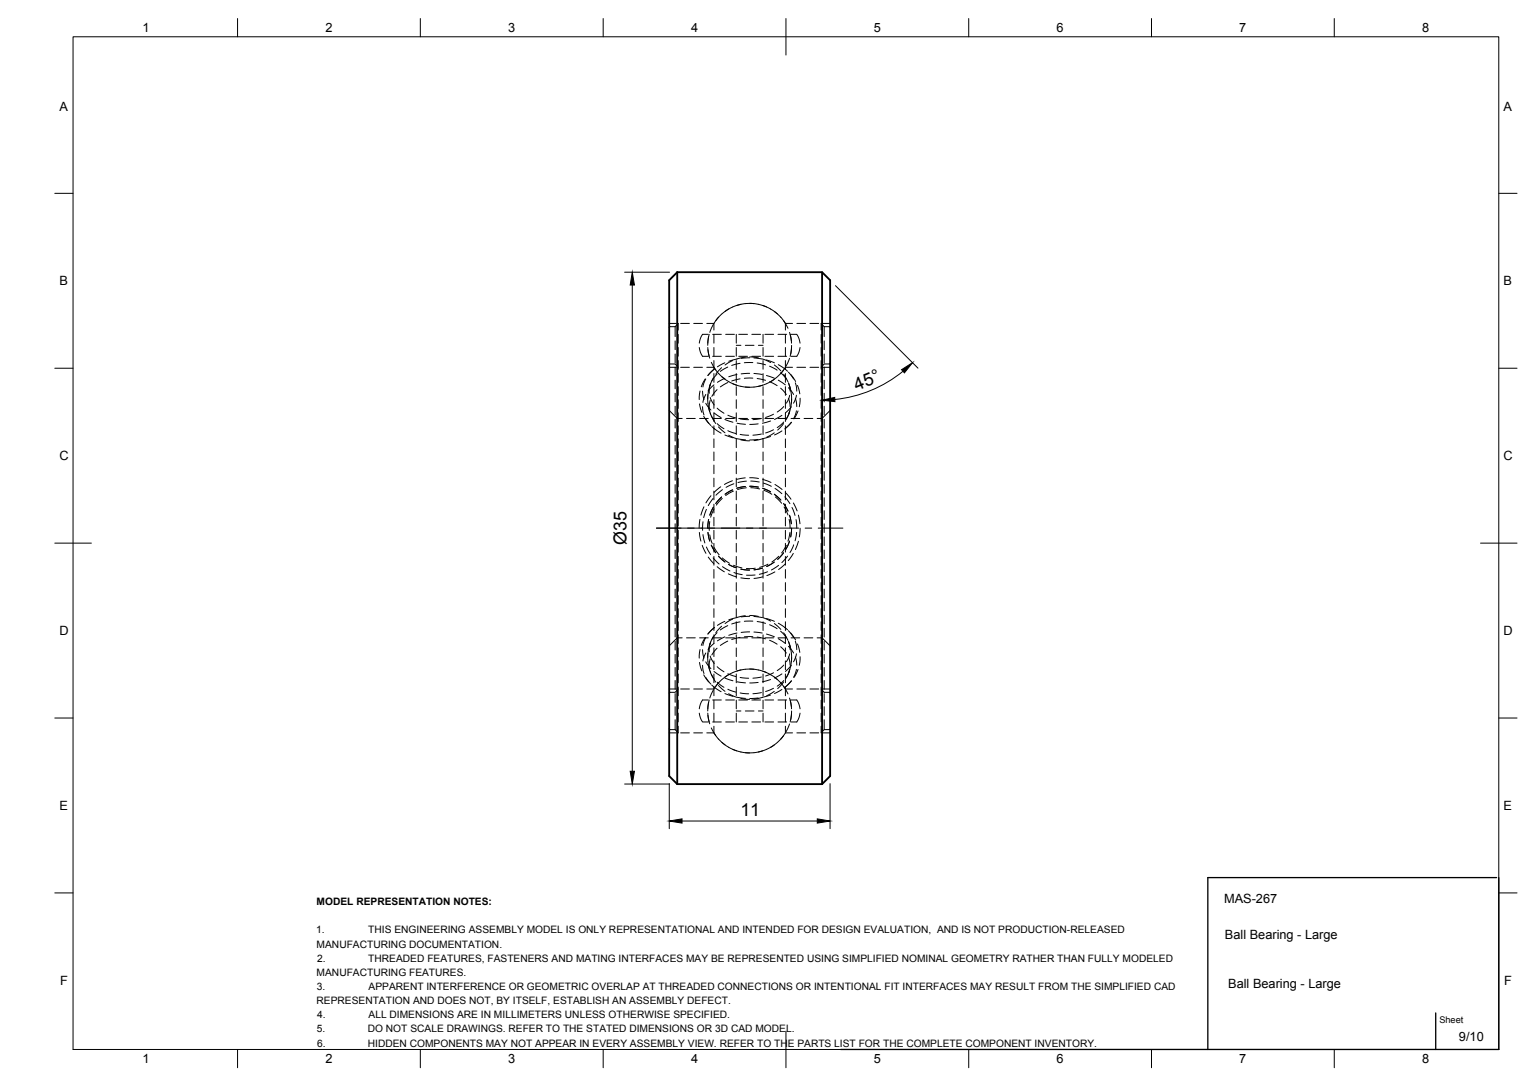
ISO-10303-21;
HEADER;
/* Generated by software containing ST-Developer
 * from STEP Tools, Inc. (www.steptools.com) 
 */

FILE_DESCRIPTION(
/* description */ (''),
/* implementation_level */ '2;1');

FILE_NAME(
/* name */ 'Ball Bearing - Large.step',
/* time_stamp */ '2026-10-12T15:29:24-07:00',
/* author */ (''),
/* organization */ (''),
/* preprocessor_version */ 'ST-DEVELOPER v20.2',
/* originating_system */ 'Autodesk Translation Framework v15.15.0.0',
/* authorisation */ '');

FILE_SCHEMA (('AUTOMOTIVE_DESIGN { 1 0 10303 214 3 1 1 }'));
ENDSEC;

DATA;
#10=MECHANICAL_DESIGN_GEOMETRIC_PRESENTATION_REPRESENTATION('',(#198,#199,#200,#201,#202,#203,#204,#205,#206,#207,#208,#209,#210,#211,#212,#213,#214,#215,#216,#217,#218),#9496);
#116=CONICAL_SURFACE('',#5581,8.04999999999999,0.78539816339744);
#117=CONICAL_SURFACE('',#5587,7.5,0.78539816339744);
#118=CONICAL_SURFACE('',#5597,16.95,0.785398163397447);
#119=CONICAL_SURFACE('',#5608,17.5,0.785398163397446);
#120=CONICAL_SURFACE('',#5730,14.,0.835033387742089);
#121=CONICAL_SURFACE('',#5732,11.225,0.835033387742081);
#122=CONICAL_SURFACE('',#5749,11.,0.835033387742083);
#123=CONICAL_SURFACE('',#5751,13.775,0.835033387742092);
#131=TOROIDAL_SURFACE('',#5577,12.5,2.86797988869785);
#132=TOROIDAL_SURFACE('',#5603,12.5,2.86797988869785);
#133=TOROIDAL_SURFACE('',#5629,2.10186832938358,1.34926506255229);
#134=TOROIDAL_SURFACE('',#5639,2.10186832938358,1.34926506255229);
#135=TOROIDAL_SURFACE('',#5649,2.10186832938358,1.34926506255229);
#136=TOROIDAL_SURFACE('',#5659,2.10186832938358,1.34926506255229);
#137=TOROIDAL_SURFACE('',#5669,2.10186832938358,1.34926506255229);
#138=TOROIDAL_SURFACE('',#5679,2.10186832938358,1.34926506255229);
#139=TOROIDAL_SURFACE('',#5689,2.10186832938358,1.34926506255229);
#140=TOROIDAL_SURFACE('',#5699,2.10186832938358,1.34926506255229);
#141=TOROIDAL_SURFACE('',#5717,11.2861111111111,0.0611111111111111);
#142=TOROIDAL_SURFACE('',#5722,13.7138888888889,0.0611111111111111);
#143=TOROIDAL_SURFACE('',#5738,13.7138888888889,0.061111111111111);
#144=TOROIDAL_SURFACE('',#5742,11.2861111111111,0.061111111111111);
#152=SHAPE_REPRESENTATION_RELATIONSHIP('SRR','None',#9546,#161);
#161=ADVANCED_BREP_SHAPE_REPRESENTATION('',(#255,#256,#257,#258,#259,#260,
#261,#262,#263,#264,#265,#266,#267,#268,#269,#270,#271,#272,#273,#274,#275),
#9494);
#198=STYLED_ITEM('',(#9594),#255);
#199=STYLED_ITEM('',(#9594),#256);
#200=STYLED_ITEM('',(#9594),#257);
#201=STYLED_ITEM('',(#9594),#258);
#202=STYLED_ITEM('',(#9594),#259);
#203=STYLED_ITEM('',(#9594),#260);
#204=STYLED_ITEM('',(#9594),#261);
#205=STYLED_ITEM('',(#9594),#262);
#206=STYLED_ITEM('',(#9594),#263);
#207=STYLED_ITEM('',(#9594),#264);
#208=STYLED_ITEM('',(#9594),#265);
#209=STYLED_ITEM('',(#9594),#266);
#210=STYLED_ITEM('',(#9594),#267);
#211=STYLED_ITEM('',(#9594),#268);
#212=STYLED_ITEM('',(#9594),#269);
#213=STYLED_ITEM('',(#9594),#270);
#214=STYLED_ITEM('',(#9594),#271);
#215=STYLED_ITEM('',(#9594),#272);
#216=STYLED_ITEM('',(#9594),#273);
#217=STYLED_ITEM('',(#9594),#274);
#218=STYLED_ITEM('',(#9594),#275);
#255=MANIFOLD_SOLID_BREP('Body1',#5000);
#256=MANIFOLD_SOLID_BREP('Body2',#5001);
#257=MANIFOLD_SOLID_BREP('Body3',#5002);
#258=MANIFOLD_SOLID_BREP('Body4',#5003);
#259=MANIFOLD_SOLID_BREP('Body5',#5004);
#260=MANIFOLD_SOLID_BREP('Body6',#5005);
#261=MANIFOLD_SOLID_BREP('Body7',#5006);
#262=MANIFOLD_SOLID_BREP('Body8',#5007);
#263=MANIFOLD_SOLID_BREP('Body9',#5008);
#264=MANIFOLD_SOLID_BREP('Body10',#5009);
#265=MANIFOLD_SOLID_BREP('Body11',#5010);
#266=MANIFOLD_SOLID_BREP('Body12',#5011);
#267=MANIFOLD_SOLID_BREP('Body13',#5012);
#268=MANIFOLD_SOLID_BREP('Body14',#5013);
#269=MANIFOLD_SOLID_BREP('Body15',#5014);
#270=MANIFOLD_SOLID_BREP('Body16',#5015);
#271=MANIFOLD_SOLID_BREP('Body17',#5016);
#272=MANIFOLD_SOLID_BREP('Body18',#5017);
#273=MANIFOLD_SOLID_BREP('Body19',#5018);
#274=MANIFOLD_SOLID_BREP('Body20',#5019);
#275=MANIFOLD_SOLID_BREP('Body21',#5020);
#317=SPHERICAL_SURFACE('',#5595,2.86797988869785);
#318=SPHERICAL_SURFACE('',#5615,2.86797988869785);
#319=SPHERICAL_SURFACE('',#5617,2.86797988869785);
#320=SPHERICAL_SURFACE('',#5619,2.86797988869785);
#321=SPHERICAL_SURFACE('',#5621,2.86797988869785);
#322=SPHERICAL_SURFACE('',#5623,2.86797988869785);
#323=SPHERICAL_SURFACE('',#5625,2.86797988869785);
#324=SPHERICAL_SURFACE('',#5627,2.86797988869785);
#325=SPHERICAL_SURFACE('',#5633,2.86797988869795);
#326=SPHERICAL_SURFACE('',#5643,2.86797988869795);
#327=SPHERICAL_SURFACE('',#5653,2.86797988869795);
#328=SPHERICAL_SURFACE('',#5663,2.86797988869795);
#329=SPHERICAL_SURFACE('',#5673,2.86797988869795);
#330=SPHERICAL_SURFACE('',#5683,2.86797988869795);
#331=SPHERICAL_SURFACE('',#5693,2.86797988869795);
#332=SPHERICAL_SURFACE('',#5703,2.86797988869795);
#418=FACE_BOUND('',#1265,.T.);
#419=FACE_BOUND('',#1267,.T.);
#420=FACE_BOUND('',#1276,.T.);
#421=FACE_BOUND('',#1278,.T.);
#422=FACE_BOUND('',#1288,.T.);
#423=FACE_BOUND('',#1289,.T.);
#424=FACE_BOUND('',#1291,.T.);
#425=FACE_BOUND('',#1293,.T.);
#426=FACE_BOUND('',#1296,.T.);
#427=FACE_BOUND('',#1297,.T.);
#428=FACE_BOUND('',#1299,.T.);
#429=FACE_BOUND('',#1301,.T.);
#430=FACE_BOUND('',#1304,.T.);
#431=FACE_BOUND('',#1305,.T.);
#432=FACE_BOUND('',#1307,.T.);
#433=FACE_BOUND('',#1309,.T.);
#434=FACE_BOUND('',#1312,.T.);
#435=FACE_BOUND('',#1313,.T.);
#436=FACE_BOUND('',#1315,.T.);
#437=FACE_BOUND('',#1317,.T.);
#438=FACE_BOUND('',#1320,.T.);
#439=FACE_BOUND('',#1321,.T.);
#440=FACE_BOUND('',#1323,.T.);
#441=FACE_BOUND('',#1325,.T.);
#442=FACE_BOUND('',#1328,.T.);
#443=FACE_BOUND('',#1329,.T.);
#444=FACE_BOUND('',#1331,.T.);
#445=FACE_BOUND('',#1333,.T.);
#446=FACE_BOUND('',#1336,.T.);
#447=FACE_BOUND('',#1337,.T.);
#448=FACE_BOUND('',#1339,.T.);
#449=FACE_BOUND('',#1341,.T.);
#450=FACE_BOUND('',#1344,.T.);
#451=FACE_BOUND('',#1345,.T.);
#452=FACE_BOUND('',#1347,.T.);
#453=FACE_BOUND('',#1349,.T.);
#454=FACE_BOUND('',#1353,.T.);
#455=FACE_BOUND('',#1355,.T.);
#456=FACE_BOUND('',#1363,.T.);
#457=FACE_BOUND('',#1365,.T.);
#458=FACE_BOUND('',#1373,.T.);
#459=FACE_BOUND('',#1375,.T.);
#570=PLANE('',#5593);
#571=PLANE('',#5594);
#572=PLANE('',#5613);
#573=PLANE('',#5614);
#574=PLANE('',#5637);
#575=PLANE('',#5638);
#576=PLANE('',#5647);
#577=PLANE('',#5648);
#578=PLANE('',#5657);
#579=PLANE('',#5658);
#580=PLANE('',#5667);
#581=PLANE('',#5668);
#582=PLANE('',#5677);
#583=PLANE('',#5678);
#584=PLANE('',#5687);
#585=PLANE('',#5688);
#586=PLANE('',#5697);
#587=PLANE('',#5698);
#588=PLANE('',#5707);
#589=PLANE('',#5708);
#590=PLANE('',#5715);
#591=PLANE('',#5716);
#592=PLANE('',#5736);
#593=PLANE('',#5737);
#594=PLANE('',#5755);
#595=PLANE('',#5756);
#841=FACE_OUTER_BOUND('',#1258,.T.);
#842=FACE_OUTER_BOUND('',#1259,.T.);
#843=FACE_OUTER_BOUND('',#1260,.T.);
#844=FACE_OUTER_BOUND('',#1261,.T.);
#845=FACE_OUTER_BOUND('',#1262,.T.);
#846=FACE_OUTER_BOUND('',#1263,.T.);
#847=FACE_OUTER_BOUND('',#1264,.T.);
#848=FACE_OUTER_BOUND('',#1266,.T.);
#849=FACE_OUTER_BOUND('',#1268,.T.);
#850=FACE_OUTER_BOUND('',#1269,.T.);
#851=FACE_OUTER_BOUND('',#1270,.T.);
#852=FACE_OUTER_BOUND('',#1271,.T.);
#853=FACE_OUTER_BOUND('',#1272,.T.);
#854=FACE_OUTER_BOUND('',#1273,.T.);
#855=FACE_OUTER_BOUND('',#1274,.T.);
#856=FACE_OUTER_BOUND('',#1275,.T.);
#857=FACE_OUTER_BOUND('',#1277,.T.);
#858=FACE_OUTER_BOUND('',#1279,.T.);
#859=FACE_OUTER_BOUND('',#1280,.T.);
#860=FACE_OUTER_BOUND('',#1281,.T.);
#861=FACE_OUTER_BOUND('',#1282,.T.);
#862=FACE_OUTER_BOUND('',#1283,.T.);
#863=FACE_OUTER_BOUND('',#1284,.T.);
#864=FACE_OUTER_BOUND('',#1285,.T.);
#865=FACE_OUTER_BOUND('',#1286,.T.);
#866=FACE_OUTER_BOUND('',#1287,.T.);
#867=FACE_OUTER_BOUND('',#1290,.T.);
#868=FACE_OUTER_BOUND('',#1292,.T.);
#869=FACE_OUTER_BOUND('',#1294,.T.);
#870=FACE_OUTER_BOUND('',#1295,.T.);
#871=FACE_OUTER_BOUND('',#1298,.T.);
#872=FACE_OUTER_BOUND('',#1300,.T.);
#873=FACE_OUTER_BOUND('',#1302,.T.);
#874=FACE_OUTER_BOUND('',#1303,.T.);
#875=FACE_OUTER_BOUND('',#1306,.T.);
#876=FACE_OUTER_BOUND('',#1308,.T.);
#877=FACE_OUTER_BOUND('',#1310,.T.);
#878=FACE_OUTER_BOUND('',#1311,.T.);
#879=FACE_OUTER_BOUND('',#1314,.T.);
#880=FACE_OUTER_BOUND('',#1316,.T.);
#881=FACE_OUTER_BOUND('',#1318,.T.);
#882=FACE_OUTER_BOUND('',#1319,.T.);
#883=FACE_OUTER_BOUND('',#1322,.T.);
#884=FACE_OUTER_BOUND('',#1324,.T.);
#885=FACE_OUTER_BOUND('',#1326,.T.);
#886=FACE_OUTER_BOUND('',#1327,.T.);
#887=FACE_OUTER_BOUND('',#1330,.T.);
#888=FACE_OUTER_BOUND('',#1332,.T.);
#889=FACE_OUTER_BOUND('',#1334,.T.);
#890=FACE_OUTER_BOUND('',#1335,.T.);
#891=FACE_OUTER_BOUND('',#1338,.T.);
#892=FACE_OUTER_BOUND('',#1340,.T.);
#893=FACE_OUTER_BOUND('',#1342,.T.);
#894=FACE_OUTER_BOUND('',#1343,.T.);
#895=FACE_OUTER_BOUND('',#1346,.T.);
#896=FACE_OUTER_BOUND('',#1348,.T.);
#897=FACE_OUTER_BOUND('',#1350,.T.);
#898=FACE_OUTER_BOUND('',#1351,.T.);
#899=FACE_OUTER_BOUND('',#1352,.T.);
#900=FACE_OUTER_BOUND('',#1354,.T.);
#901=FACE_OUTER_BOUND('',#1356,.T.);
#902=FACE_OUTER_BOUND('',#1357,.T.);
#903=FACE_OUTER_BOUND('',#1358,.T.);
#904=FACE_OUTER_BOUND('',#1359,.T.);
#905=FACE_OUTER_BOUND('',#1360,.T.);
#906=FACE_OUTER_BOUND('',#1361,.T.);
#907=FACE_OUTER_BOUND('',#1362,.T.);
#908=FACE_OUTER_BOUND('',#1364,.T.);
#909=FACE_OUTER_BOUND('',#1366,.T.);
#910=FACE_OUTER_BOUND('',#1367,.T.);
#911=FACE_OUTER_BOUND('',#1368,.T.);
#912=FACE_OUTER_BOUND('',#1369,.T.);
#913=FACE_OUTER_BOUND('',#1370,.T.);
#914=FACE_OUTER_BOUND('',#1371,.T.);
#915=FACE_OUTER_BOUND('',#1372,.T.);
#916=FACE_OUTER_BOUND('',#1374,.T.);
#1258=EDGE_LOOP('',(#4071,#4072,#4073,#4074));
#1259=EDGE_LOOP('',(#4075,#4076,#4077,#4078));
#1260=EDGE_LOOP('',(#4079,#4080,#4081,#4082,#4083));
#1261=EDGE_LOOP('',(#4084,#4085,#4086,#4087,#4088));
#1262=EDGE_LOOP('',(#4089,#4090,#4091,#4092));
#1263=EDGE_LOOP('',(#4093,#4094,#4095,#4096));
#1264=EDGE_LOOP('',(#4097));
#1265=EDGE_LOOP('',(#4098));
#1266=EDGE_LOOP('',(#4099));
#1267=EDGE_LOOP('',(#4100));
#1268=EDGE_LOOP('',(#4101,#4102));
#1269=EDGE_LOOP('',(#4103,#4104,#4105,#4106));
#1270=EDGE_LOOP('',(#4107,#4108,#4109,#4110));
#1271=EDGE_LOOP('',(#4111,#4112,#4113,#4114));
#1272=EDGE_LOOP('',(#4115,#4116,#4117,#4118));
#1273=EDGE_LOOP('',(#4119,#4120,#4121,#4122,#4123));
#1274=EDGE_LOOP('',(#4124,#4125,#4126,#4127,#4128));
#1275=EDGE_LOOP('',(#4129));
#1276=EDGE_LOOP('',(#4130));
#1277=EDGE_LOOP('',(#4131));
#1278=EDGE_LOOP('',(#4132));
#1279=EDGE_LOOP('',(#4133,#4134));
#1280=EDGE_LOOP('',(#4135,#4136));
#1281=EDGE_LOOP('',(#4137,#4138));
#1282=EDGE_LOOP('',(#4139,#4140));
#1283=EDGE_LOOP('',(#4141,#4142));
#1284=EDGE_LOOP('',(#4143,#4144));
#1285=EDGE_LOOP('',(#4145,#4146));
#1286=EDGE_LOOP('',(#4147,#4148,#4149,#4150));
#1287=EDGE_LOOP('',(#4151,#4152));
#1288=EDGE_LOOP('',(#4153));
#1289=EDGE_LOOP('',(#4154));
#1290=EDGE_LOOP('',(#4155));
#1291=EDGE_LOOP('',(#4156));
#1292=EDGE_LOOP('',(#4157));
#1293=EDGE_LOOP('',(#4158));
#1294=EDGE_LOOP('',(#4159,#4160,#4161,#4162));
#1295=EDGE_LOOP('',(#4163,#4164));
#1296=EDGE_LOOP('',(#4165));
#1297=EDGE_LOOP('',(#4166));
#1298=EDGE_LOOP('',(#4167));
#1299=EDGE_LOOP('',(#4168));
#1300=EDGE_LOOP('',(#4169));
#1301=EDGE_LOOP('',(#4170));
#1302=EDGE_LOOP('',(#4171,#4172,#4173,#4174));
#1303=EDGE_LOOP('',(#4175,#4176));
#1304=EDGE_LOOP('',(#4177));
#1305=EDGE_LOOP('',(#4178));
#1306=EDGE_LOOP('',(#4179));
#1307=EDGE_LOOP('',(#4180));
#1308=EDGE_LOOP('',(#4181));
#1309=EDGE_LOOP('',(#4182));
#1310=EDGE_LOOP('',(#4183,#4184,#4185,#4186));
#1311=EDGE_LOOP('',(#4187,#4188));
#1312=EDGE_LOOP('',(#4189));
#1313=EDGE_LOOP('',(#4190));
#1314=EDGE_LOOP('',(#4191));
#1315=EDGE_LOOP('',(#4192));
#1316=EDGE_LOOP('',(#4193));
#1317=EDGE_LOOP('',(#4194));
#1318=EDGE_LOOP('',(#4195,#4196,#4197,#4198));
#1319=EDGE_LOOP('',(#4199,#4200));
#1320=EDGE_LOOP('',(#4201));
#1321=EDGE_LOOP('',(#4202));
#1322=EDGE_LOOP('',(#4203));
#1323=EDGE_LOOP('',(#4204));
#1324=EDGE_LOOP('',(#4205));
#1325=EDGE_LOOP('',(#4206));
#1326=EDGE_LOOP('',(#4207,#4208,#4209,#4210));
#1327=EDGE_LOOP('',(#4211,#4212));
#1328=EDGE_LOOP('',(#4213));
#1329=EDGE_LOOP('',(#4214));
#1330=EDGE_LOOP('',(#4215));
#1331=EDGE_LOOP('',(#4216));
#1332=EDGE_LOOP('',(#4217));
#1333=EDGE_LOOP('',(#4218));
#1334=EDGE_LOOP('',(#4219,#4220,#4221,#4222));
#1335=EDGE_LOOP('',(#4223,#4224));
#1336=EDGE_LOOP('',(#4225));
#1337=EDGE_LOOP('',(#4226));
#1338=EDGE_LOOP('',(#4227));
#1339=EDGE_LOOP('',(#4228));
#1340=EDGE_LOOP('',(#4229));
#1341=EDGE_LOOP('',(#4230));
#1342=EDGE_LOOP('',(#4231,#4232,#4233,#4234));
#1343=EDGE_LOOP('',(#4235,#4236));
#1344=EDGE_LOOP('',(#4237));
#1345=EDGE_LOOP('',(#4238));
#1346=EDGE_LOOP('',(#4239));
#1347=EDGE_LOOP('',(#4240));
#1348=EDGE_LOOP('',(#4241));
#1349=EDGE_LOOP('',(#4242));
#1350=EDGE_LOOP('',(#4243,#4244,#4245,#4246));
#1351=EDGE_LOOP('',(#4247,#4248,#4249,#4250));
#1352=EDGE_LOOP('',(#4251));
#1353=EDGE_LOOP('',(#4252));
#1354=EDGE_LOOP('',(#4253));
#1355=EDGE_LOOP('',(#4254));
#1356=EDGE_LOOP('',(#4255,#4256,#4257,#4258,#4259));
#1357=EDGE_LOOP('',(#4260,#4261,#4262,#4263,#4264));
#1358=EDGE_LOOP('',(#4265,#4266,#4267,#4268,#4269,#4270));
#1359=EDGE_LOOP('',(#4271,#4272,#4273,#4274,#4275));
#1360=EDGE_LOOP('',(#4276,#4277,#4278,#4279));
#1361=EDGE_LOOP('',(#4280,#4281,#4282,#4283,#4284));
#1362=EDGE_LOOP('',(#4285));
#1363=EDGE_LOOP('',(#4286));
#1364=EDGE_LOOP('',(#4287));
#1365=EDGE_LOOP('',(#4288));
#1366=EDGE_LOOP('',(#4289,#4290,#4291,#4292));
#1367=EDGE_LOOP('',(#4293,#4294,#4295,#4296));
#1368=EDGE_LOOP('',(#4297,#4298,#4299,#4300,#4301));
#1369=EDGE_LOOP('',(#4302,#4303,#4304,#4305,#4306));
#1370=EDGE_LOOP('',(#4307,#4308,#4309,#4310));
#1371=EDGE_LOOP('',(#4311,#4312,#4313,#4314));
#1372=EDGE_LOOP('',(#4315));
#1373=EDGE_LOOP('',(#4316));
#1374=EDGE_LOOP('',(#4317));
#1375=EDGE_LOOP('',(#4318));
#1569=LINE('',#8661,#1806);
#1570=LINE('',#8668,#1807);
#1571=LINE('',#8671,#1808);
#1572=LINE('',#8675,#1809);
#1573=LINE('',#8680,#1810);
#1574=LINE('',#8691,#1811);
#1575=LINE('',#8697,#1812);
#1576=LINE('',#8705,#1813);
#1577=LINE('',#8712,#1814);
#1578=LINE('',#8716,#1815);
#1579=LINE('',#8879,#1816);
#1580=LINE('',#8885,#1817);
#1581=LINE('',#8907,#1818);
#1582=LINE('',#8914,#1819);
#1583=LINE('',#8919,#1820);
#1584=LINE('',#8922,#1821);
#1585=LINE('',#8939,#1822);
#1586=LINE('',#8946,#1823);
#1587=LINE('',#8951,#1824);
#1588=LINE('',#8954,#1825);
#1806=VECTOR('',#6882,8.04999999999999);
#1807=VECTOR('',#6891,7.5);
#1808=VECTOR('',#6894,7.5);
#1809=VECTOR('',#6899,11.);
#1810=VECTOR('',#6906,11.);
#1811=VECTOR('',#6919,16.95);
#1812=VECTOR('',#6926,14.);
#1813=VECTOR('',#6937,14.);
#1814=VECTOR('',#6944,17.5);
#1815=VECTOR('',#6951,17.5);
#1816=VECTOR('',#7148,12.5);
#1817=VECTOR('',#7155,13.25);
#1818=VECTOR('',#7184,13.775);
#1819=VECTOR('',#7193,14.);
#1820=VECTOR('',#7198,11.225);
#1821=VECTOR('',#7203,11.225);
#1822=VECTOR('',#7226,11.225);
#1823=VECTOR('',#7235,11.);
#1824=VECTOR('',#7240,13.775);
#1825=VECTOR('',#7245,13.775);
#2146=CIRCLE('',#5578,11.);
#2147=CIRCLE('',#5579,2.86797988869785);
#2148=CIRCLE('',#5580,11.);
#2149=CIRCLE('',#5582,7.5);
#2150=CIRCLE('',#5583,8.04999999999999);
#2151=CIRCLE('',#5585,7.5);
#2152=CIRCLE('',#5586,7.5);
#2153=CIRCLE('',#5588,8.04999999999999);
#2154=CIRCLE('',#5590,11.);
#2155=CIRCLE('',#5592,11.);
#2156=CIRCLE('',#5596,2.86797988869785);
#2157=CIRCLE('',#5598,17.5);
#2158=CIRCLE('',#5599,16.95);
#2159=CIRCLE('',#5601,14.);
#2160=CIRCLE('',#5602,14.);
#2161=CIRCLE('',#5604,2.86797988869785);
#2162=CIRCLE('',#5605,14.);
#2163=CIRCLE('',#5607,14.);
#2164=CIRCLE('',#5609,17.5);
#2165=CIRCLE('',#5610,16.95);
#2166=CIRCLE('',#5611,17.5);
#2167=CIRCLE('',#5616,2.86797988869785);
#2168=CIRCLE('',#5618,2.86797988869785);
#2169=CIRCLE('',#5620,2.86797988869785);
#2170=CIRCLE('',#5622,2.86797988869785);
#2171=CIRCLE('',#5624,2.86797988869785);
#2172=CIRCLE('',#5626,2.86797988869785);
#2173=CIRCLE('',#5628,2.86797988869785);
#2174=CIRCLE('',#5630,3.22348154659542);
#2175=CIRCLE('',#5631,1.34926506255229);
#2176=CIRCLE('',#5632,3.22348154659542);
#2177=CIRCLE('',#5634,2.86797988869795);
#2178=CIRCLE('',#5635,2.7681778559145);
#2179=CIRCLE('',#5636,2.7681778559145);
#2180=CIRCLE('',#5640,3.22348154659542);
#2181=CIRCLE('',#5641,1.34926506255229);
#2182=CIRCLE('',#5642,3.22348154659542);
#2183=CIRCLE('',#5644,2.86797988869795);
#2184=CIRCLE('',#5645,2.7681778559145);
#2185=CIRCLE('',#5646,2.7681778559145);
#2186=CIRCLE('',#5650,3.22348154659542);
#2187=CIRCLE('',#5651,1.34926506255229);
#2188=CIRCLE('',#5652,3.22348154659542);
#2189=CIRCLE('',#5654,2.86797988869795);
#2190=CIRCLE('',#5655,2.7681778559145);
#2191=CIRCLE('',#5656,2.7681778559145);
#2192=CIRCLE('',#5660,3.22348154659542);
#2193=CIRCLE('',#5661,1.34926506255229);
#2194=CIRCLE('',#5662,3.22348154659542);
#2195=CIRCLE('',#5664,2.86797988869795);
#2196=CIRCLE('',#5665,2.7681778559145);
#2197=CIRCLE('',#5666,2.7681778559145);
#2198=CIRCLE('',#5670,3.22348154659542);
#2199=CIRCLE('',#5671,1.34926506255229);
#2200=CIRCLE('',#5672,3.22348154659542);
#2201=CIRCLE('',#5674,2.86797988869795);
#2202=CIRCLE('',#5675,2.7681778559145);
#2203=CIRCLE('',#5676,2.7681778559145);
#2204=CIRCLE('',#5680,3.22348154659542);
#2205=CIRCLE('',#5681,1.34926506255229);
#2206=CIRCLE('',#5682,3.22348154659542);
#2207=CIRCLE('',#5684,2.86797988869795);
#2208=CIRCLE('',#5685,2.7681778559145);
#2209=CIRCLE('',#5686,2.7681778559145);
#2210=CIRCLE('',#5690,3.22348154659542);
#2211=CIRCLE('',#5691,1.34926506255229);
#2212=CIRCLE('',#5692,3.22348154659542);
#2213=CIRCLE('',#5694,2.86797988869795);
#2214=CIRCLE('',#5695,2.7681778559145);
#2215=CIRCLE('',#5696,2.7681778559145);
#2216=CIRCLE('',#5700,3.22348154659542);
#2217=CIRCLE('',#5701,1.34926506255229);
#2218=CIRCLE('',#5702,3.22348154659542);
#2219=CIRCLE('',#5704,2.86797988869795);
#2220=CIRCLE('',#5705,2.7681778559145);
#2221=CIRCLE('',#5706,2.7681778559145);
#2222=CIRCLE('',#5710,12.5);
#2223=CIRCLE('',#5711,12.5);
#2224=CIRCLE('',#5713,13.25);
#2225=CIRCLE('',#5714,13.25);
#2226=CIRCLE('',#5718,11.2861111111111);
#2227=CIRCLE('',#5719,0.0611111111111111);
#2228=CIRCLE('',#5720,11.225);
#2229=CIRCLE('',#5721,11.225);
#2230=CIRCLE('',#5723,13.775);
#2231=CIRCLE('',#5724,13.775);
#2232=CIRCLE('',#5725,0.0611111111111111);
#2233=CIRCLE('',#5726,13.7138888888889);
#2234=CIRCLE('',#5728,13.775);
#2235=CIRCLE('',#5729,13.775);
#2236=CIRCLE('',#5731,14.);
#2237=CIRCLE('',#5733,11.);
#2238=CIRCLE('',#5734,11.225);
#2239=CIRCLE('',#5739,13.775);
#2240=CIRCLE('',#5740,0.061111111111111);
#2241=CIRCLE('',#5741,13.7138888888889);
#2242=CIRCLE('',#5743,11.2861111111111);
#2243=CIRCLE('',#5744,0.061111111111111);
#2244=CIRCLE('',#5745,11.225);
#2245=CIRCLE('',#5747,11.225);
#2246=CIRCLE('',#5748,11.225);
#2247=CIRCLE('',#5750,11.);
#2248=CIRCLE('',#5752,14.);
#2249=CIRCLE('',#5753,13.775);
#2531=VERTEX_POINT('',#8652);
#2532=VERTEX_POINT('',#8654);
#2533=VERTEX_POINT('',#8658);
#2534=VERTEX_POINT('',#8660);
#2535=VERTEX_POINT('',#8664);
#2536=VERTEX_POINT('',#8665);
#2537=VERTEX_POINT('',#8670);
#2538=VERTEX_POINT('',#8674);
#2539=VERTEX_POINT('',#8678);
#2540=VERTEX_POINT('',#8684);
#2541=VERTEX_POINT('',#8685);
#2542=VERTEX_POINT('',#8688);
#2543=VERTEX_POINT('',#8690);
#2544=VERTEX_POINT('',#8694);
#2545=VERTEX_POINT('',#8696);
#2546=VERTEX_POINT('',#8700);
#2547=VERTEX_POINT('',#8704);
#2548=VERTEX_POINT('',#8708);
#2549=VERTEX_POINT('',#8709);
#2550=VERTEX_POINT('',#8711);
#2551=VERTEX_POINT('',#8720);
#2552=VERTEX_POINT('',#8721);
#2553=VERTEX_POINT('',#8724);
#2554=VERTEX_POINT('',#8725);
#2555=VERTEX_POINT('',#8728);
#2556=VERTEX_POINT('',#8729);
#2557=VERTEX_POINT('',#8732);
#2558=VERTEX_POINT('',#8733);
#2559=VERTEX_POINT('',#8736);
#2560=VERTEX_POINT('',#8737);
#2561=VERTEX_POINT('',#8740);
#2562=VERTEX_POINT('',#8741);
#2563=VERTEX_POINT('',#8744);
#2564=VERTEX_POINT('',#8745);
#2565=VERTEX_POINT('',#8748);
#2566=VERTEX_POINT('',#8750);
#2567=VERTEX_POINT('',#8754);
#2568=VERTEX_POINT('',#8755);
#2569=VERTEX_POINT('',#8757);
#2570=VERTEX_POINT('',#8759);
#2571=VERTEX_POINT('',#8764);
#2572=VERTEX_POINT('',#8766);
#2573=VERTEX_POINT('',#8770);
#2574=VERTEX_POINT('',#8771);
#2575=VERTEX_POINT('',#8773);
#2576=VERTEX_POINT('',#8775);
#2577=VERTEX_POINT('',#8780);
#2578=VERTEX_POINT('',#8782);
#2579=VERTEX_POINT('',#8786);
#2580=VERTEX_POINT('',#8787);
#2581=VERTEX_POINT('',#8789);
#2582=VERTEX_POINT('',#8791);
#2583=VERTEX_POINT('',#8796);
#2584=VERTEX_POINT('',#8798);
#2585=VERTEX_POINT('',#8802);
#2586=VERTEX_POINT('',#8803);
#2587=VERTEX_POINT('',#8805);
#2588=VERTEX_POINT('',#8807);
#2589=VERTEX_POINT('',#8812);
#2590=VERTEX_POINT('',#8814);
#2591=VERTEX_POINT('',#8818);
#2592=VERTEX_POINT('',#8819);
#2593=VERTEX_POINT('',#8821);
#2594=VERTEX_POINT('',#8823);
#2595=VERTEX_POINT('',#8828);
#2596=VERTEX_POINT('',#8830);
#2597=VERTEX_POINT('',#8834);
#2598=VERTEX_POINT('',#8835);
#2599=VERTEX_POINT('',#8837);
#2600=VERTEX_POINT('',#8839);
#2601=VERTEX_POINT('',#8844);
#2602=VERTEX_POINT('',#8846);
#2603=VERTEX_POINT('',#8850);
#2604=VERTEX_POINT('',#8851);
#2605=VERTEX_POINT('',#8853);
#2606=VERTEX_POINT('',#8855);
#2607=VERTEX_POINT('',#8860);
#2608=VERTEX_POINT('',#8862);
#2609=VERTEX_POINT('',#8866);
#2610=VERTEX_POINT('',#8867);
#2611=VERTEX_POINT('',#8869);
#2612=VERTEX_POINT('',#8871);
#2613=VERTEX_POINT('',#8876);
#2614=VERTEX_POINT('',#8878);
#2615=VERTEX_POINT('',#8882);
#2616=VERTEX_POINT('',#8884);
#2617=VERTEX_POINT('',#8890);
#2618=VERTEX_POINT('',#8892);
#2619=VERTEX_POINT('',#8894);
#2620=VERTEX_POINT('',#8898);
#2621=VERTEX_POINT('',#8899);
#2622=VERTEX_POINT('',#8902);
#2623=VERTEX_POINT('',#8906);
#2624=VERTEX_POINT('',#8908);
#2625=VERTEX_POINT('',#8912);
#2626=VERTEX_POINT('',#8916);
#2627=VERTEX_POINT('',#8918);
#2628=VERTEX_POINT('',#8926);
#2629=VERTEX_POINT('',#8928);
#2630=VERTEX_POINT('',#8932);
#2631=VERTEX_POINT('',#8934);
#2632=VERTEX_POINT('',#8938);
#2633=VERTEX_POINT('',#8940);
#2634=VERTEX_POINT('',#8944);
#2635=VERTEX_POINT('',#8948);
#2636=VERTEX_POINT('',#8950);
#3088=EDGE_CURVE('',#2531,#2531,#2146,.T.);
#3089=EDGE_CURVE('',#2531,#2532,#2147,.T.);
#3090=EDGE_CURVE('',#2532,#2532,#2148,.T.);
#3091=EDGE_CURVE('',#2533,#2533,#2149,.T.);
#3092=EDGE_CURVE('',#2533,#2534,#1569,.T.);
#3093=EDGE_CURVE('',#2534,#2534,#2150,.T.);
#3094=EDGE_CURVE('',#2535,#2536,#2151,.T.);
#3095=EDGE_CURVE('',#2536,#2535,#2152,.T.);
#3096=EDGE_CURVE('',#2536,#2533,#1570,.T.);
#3097=EDGE_CURVE('',#2535,#2537,#1571,.T.);
#3098=EDGE_CURVE('',#2537,#2537,#2153,.T.);
#3099=EDGE_CURVE('',#2532,#2538,#1572,.T.);
#3100=EDGE_CURVE('',#2538,#2538,#2154,.T.);
#3101=EDGE_CURVE('',#2539,#2539,#2155,.T.);
#3102=EDGE_CURVE('',#2539,#2531,#1573,.T.);
#3103=EDGE_CURVE('',#2540,#2541,#2156,.T.);
#3104=EDGE_CURVE('',#2542,#2542,#2157,.T.);
#3105=EDGE_CURVE('',#2542,#2543,#1574,.T.);
#3106=EDGE_CURVE('',#2543,#2543,#2158,.T.);
#3107=EDGE_CURVE('',#2544,#2544,#2159,.T.);
#3108=EDGE_CURVE('',#2544,#2545,#1575,.T.);
#3109=EDGE_CURVE('',#2545,#2545,#2160,.T.);
#3110=EDGE_CURVE('',#2545,#2546,#2161,.T.);
#3111=EDGE_CURVE('',#2546,#2546,#2162,.T.);
#3112=EDGE_CURVE('',#2546,#2547,#1576,.T.);
#3113=EDGE_CURVE('',#2547,#2547,#2163,.T.);
#3114=EDGE_CURVE('',#2548,#2549,#2164,.T.);
#3115=EDGE_CURVE('',#2549,#2550,#1577,.T.);
#3116=EDGE_CURVE('',#2550,#2550,#2165,.T.);
#3117=EDGE_CURVE('',#2549,#2548,#2166,.T.);
#3118=EDGE_CURVE('',#2548,#2542,#1578,.T.);
#3119=EDGE_CURVE('',#2551,#2552,#2167,.T.);
#3120=EDGE_CURVE('',#2553,#2554,#2168,.T.);
#3121=EDGE_CURVE('',#2555,#2556,#2169,.T.);
#3122=EDGE_CURVE('',#2557,#2558,#2170,.T.);
#3123=EDGE_CURVE('',#2559,#2560,#2171,.T.);
#3124=EDGE_CURVE('',#2561,#2562,#2172,.T.);
#3125=EDGE_CURVE('',#2563,#2564,#2173,.T.);
#3126=EDGE_CURVE('',#2565,#2565,#2174,.T.);
#3127=EDGE_CURVE('',#2565,#2566,#2175,.T.);
#3128=EDGE_CURVE('',#2566,#2566,#2176,.T.);
#3129=EDGE_CURVE('',#2567,#2568,#2177,.T.);
#3130=EDGE_CURVE('',#2569,#2569,#2178,.T.);
#3131=EDGE_CURVE('',#2570,#2570,#2179,.T.);
#3132=EDGE_CURVE('',#2571,#2571,#2180,.T.);
#3133=EDGE_CURVE('',#2571,#2572,#2181,.T.);
#3134=EDGE_CURVE('',#2572,#2572,#2182,.T.);
#3135=EDGE_CURVE('',#2573,#2574,#2183,.T.);
#3136=EDGE_CURVE('',#2575,#2575,#2184,.T.);
#3137=EDGE_CURVE('',#2576,#2576,#2185,.T.);
#3138=EDGE_CURVE('',#2577,#2577,#2186,.T.);
#3139=EDGE_CURVE('',#2577,#2578,#2187,.T.);
#3140=EDGE_CURVE('',#2578,#2578,#2188,.T.);
#3141=EDGE_CURVE('',#2579,#2580,#2189,.T.);
#3142=EDGE_CURVE('',#2581,#2581,#2190,.T.);
#3143=EDGE_CURVE('',#2582,#2582,#2191,.T.);
#3144=EDGE_CURVE('',#2583,#2583,#2192,.T.);
#3145=EDGE_CURVE('',#2583,#2584,#2193,.T.);
#3146=EDGE_CURVE('',#2584,#2584,#2194,.T.);
#3147=EDGE_CURVE('',#2585,#2586,#2195,.T.);
#3148=EDGE_CURVE('',#2587,#2587,#2196,.T.);
#3149=EDGE_CURVE('',#2588,#2588,#2197,.T.);
#3150=EDGE_CURVE('',#2589,#2589,#2198,.T.);
#3151=EDGE_CURVE('',#2589,#2590,#2199,.T.);
#3152=EDGE_CURVE('',#2590,#2590,#2200,.T.);
#3153=EDGE_CURVE('',#2591,#2592,#2201,.T.);
#3154=EDGE_CURVE('',#2593,#2593,#2202,.T.);
#3155=EDGE_CURVE('',#2594,#2594,#2203,.T.);
#3156=EDGE_CURVE('',#2595,#2595,#2204,.T.);
#3157=EDGE_CURVE('',#2595,#2596,#2205,.T.);
#3158=EDGE_CURVE('',#2596,#2596,#2206,.T.);
#3159=EDGE_CURVE('',#2597,#2598,#2207,.T.);
#3160=EDGE_CURVE('',#2599,#2599,#2208,.T.);
#3161=EDGE_CURVE('',#2600,#2600,#2209,.T.);
#3162=EDGE_CURVE('',#2601,#2601,#2210,.T.);
#3163=EDGE_CURVE('',#2601,#2602,#2211,.T.);
#3164=EDGE_CURVE('',#2602,#2602,#2212,.T.);
#3165=EDGE_CURVE('',#2603,#2604,#2213,.T.);
#3166=EDGE_CURVE('',#2605,#2605,#2214,.T.);
#3167=EDGE_CURVE('',#2606,#2606,#2215,.T.);
#3168=EDGE_CURVE('',#2607,#2607,#2216,.T.);
#3169=EDGE_CURVE('',#2607,#2608,#2217,.T.);
#3170=EDGE_CURVE('',#2608,#2608,#2218,.T.);
#3171=EDGE_CURVE('',#2609,#2610,#2219,.T.);
#3172=EDGE_CURVE('',#2611,#2611,#2220,.T.);
#3173=EDGE_CURVE('',#2612,#2612,#2221,.T.);
#3174=EDGE_CURVE('',#2613,#2613,#2222,.T.);
#3175=EDGE_CURVE('',#2613,#2614,#1579,.T.);
#3176=EDGE_CURVE('',#2614,#2614,#2223,.T.);
#3177=EDGE_CURVE('',#2615,#2615,#2224,.T.);
#3178=EDGE_CURVE('',#2615,#2616,#1580,.T.);
#3179=EDGE_CURVE('',#2616,#2616,#2225,.T.);
#3180=EDGE_CURVE('',#2617,#2617,#2226,.T.);
#3181=EDGE_CURVE('',#2617,#2618,#2227,.T.);
#3182=EDGE_CURVE('',#2619,#2618,#2228,.T.);
#3183=EDGE_CURVE('',#2618,#2619,#2229,.T.);
#3184=EDGE_CURVE('',#2620,#2621,#2230,.T.);
#3185=EDGE_CURVE('',#2621,#2620,#2231,.T.);
#3186=EDGE_CURVE('',#2621,#2622,#2232,.T.);
#3187=EDGE_CURVE('',#2622,#2622,#2233,.T.);
#3188=EDGE_CURVE('',#2620,#2623,#1581,.T.);
#3189=EDGE_CURVE('',#2623,#2624,#2234,.T.);
#3190=EDGE_CURVE('',#2624,#2623,#2235,.T.);
#3191=EDGE_CURVE('',#2625,#2625,#2236,.T.);
#3192=EDGE_CURVE('',#2625,#2624,#1582,.T.);
#3193=EDGE_CURVE('',#2626,#2626,#2237,.T.);
#3194=EDGE_CURVE('',#2626,#2627,#1583,.T.);
#3195=EDGE_CURVE('',#2627,#2627,#2238,.T.);
#3196=EDGE_CURVE('',#2627,#2619,#1584,.T.);
#3197=EDGE_CURVE('',#2628,#2628,#2239,.T.);
#3198=EDGE_CURVE('',#2628,#2629,#2240,.T.);
#3199=EDGE_CURVE('',#2629,#2629,#2241,.T.);
#3200=EDGE_CURVE('',#2630,#2630,#2242,.T.);
#3201=EDGE_CURVE('',#2630,#2631,#2243,.T.);
#3202=EDGE_CURVE('',#2631,#2631,#2244,.T.);
#3203=EDGE_CURVE('',#2631,#2632,#1585,.T.);
#3204=EDGE_CURVE('',#2632,#2633,#2245,.T.);
#3205=EDGE_CURVE('',#2633,#2632,#2246,.T.);
#3206=EDGE_CURVE('',#2634,#2634,#2247,.T.);
#3207=EDGE_CURVE('',#2634,#2633,#1586,.T.);
#3208=EDGE_CURVE('',#2635,#2635,#2248,.T.);
#3209=EDGE_CURVE('',#2635,#2636,#1587,.T.);
#3210=EDGE_CURVE('',#2636,#2636,#2249,.T.);
#3211=EDGE_CURVE('',#2636,#2628,#1588,.T.);
#4071=ORIENTED_EDGE('',*,*,#3088,.F.);
#4072=ORIENTED_EDGE('',*,*,#3089,.T.);
#4073=ORIENTED_EDGE('',*,*,#3090,.T.);
#4074=ORIENTED_EDGE('',*,*,#3089,.F.);
#4075=ORIENTED_EDGE('',*,*,#3091,.F.);
#4076=ORIENTED_EDGE('',*,*,#3092,.T.);
#4077=ORIENTED_EDGE('',*,*,#3093,.T.);
#4078=ORIENTED_EDGE('',*,*,#3092,.F.);
#4079=ORIENTED_EDGE('',*,*,#3094,.F.);
#4080=ORIENTED_EDGE('',*,*,#3095,.F.);
#4081=ORIENTED_EDGE('',*,*,#3096,.T.);
#4082=ORIENTED_EDGE('',*,*,#3091,.T.);
#4083=ORIENTED_EDGE('',*,*,#3096,.F.);
#4084=ORIENTED_EDGE('',*,*,#3094,.T.);
#4085=ORIENTED_EDGE('',*,*,#3095,.T.);
#4086=ORIENTED_EDGE('',*,*,#3097,.T.);
#4087=ORIENTED_EDGE('',*,*,#3098,.F.);
#4088=ORIENTED_EDGE('',*,*,#3097,.F.);
#4089=ORIENTED_EDGE('',*,*,#3090,.F.);
#4090=ORIENTED_EDGE('',*,*,#3099,.T.);
#4091=ORIENTED_EDGE('',*,*,#3100,.T.);
#4092=ORIENTED_EDGE('',*,*,#3099,.F.);
#4093=ORIENTED_EDGE('',*,*,#3101,.F.);
#4094=ORIENTED_EDGE('',*,*,#3102,.T.);
#4095=ORIENTED_EDGE('',*,*,#3088,.T.);
#4096=ORIENTED_EDGE('',*,*,#3102,.F.);
#4097=ORIENTED_EDGE('',*,*,#3101,.T.);
#4098=ORIENTED_EDGE('',*,*,#3093,.F.);
#4099=ORIENTED_EDGE('',*,*,#3100,.F.);
#4100=ORIENTED_EDGE('',*,*,#3098,.T.);
#4101=ORIENTED_EDGE('',*,*,#3103,.T.);
#4102=ORIENTED_EDGE('',*,*,#3103,.F.);
#4103=ORIENTED_EDGE('',*,*,#3104,.F.);
#4104=ORIENTED_EDGE('',*,*,#3105,.T.);
#4105=ORIENTED_EDGE('',*,*,#3106,.T.);
#4106=ORIENTED_EDGE('',*,*,#3105,.F.);
#4107=ORIENTED_EDGE('',*,*,#3107,.F.);
#4108=ORIENTED_EDGE('',*,*,#3108,.T.);
#4109=ORIENTED_EDGE('',*,*,#3109,.T.);
#4110=ORIENTED_EDGE('',*,*,#3108,.F.);
#4111=ORIENTED_EDGE('',*,*,#3109,.F.);
#4112=ORIENTED_EDGE('',*,*,#3110,.T.);
#4113=ORIENTED_EDGE('',*,*,#3111,.T.);
#4114=ORIENTED_EDGE('',*,*,#3110,.F.);
#4115=ORIENTED_EDGE('',*,*,#3111,.F.);
#4116=ORIENTED_EDGE('',*,*,#3112,.T.);
#4117=ORIENTED_EDGE('',*,*,#3113,.T.);
#4118=ORIENTED_EDGE('',*,*,#3112,.F.);
#4119=ORIENTED_EDGE('',*,*,#3114,.T.);
#4120=ORIENTED_EDGE('',*,*,#3115,.T.);
#4121=ORIENTED_EDGE('',*,*,#3116,.F.);
#4122=ORIENTED_EDGE('',*,*,#3115,.F.);
#4123=ORIENTED_EDGE('',*,*,#3117,.T.);
#4124=ORIENTED_EDGE('',*,*,#3114,.F.);
#4125=ORIENTED_EDGE('',*,*,#3118,.T.);
#4126=ORIENTED_EDGE('',*,*,#3104,.T.);
#4127=ORIENTED_EDGE('',*,*,#3118,.F.);
#4128=ORIENTED_EDGE('',*,*,#3117,.F.);
#4129=ORIENTED_EDGE('',*,*,#3116,.T.);
#4130=ORIENTED_EDGE('',*,*,#3113,.F.);
#4131=ORIENTED_EDGE('',*,*,#3106,.F.);
#4132=ORIENTED_EDGE('',*,*,#3107,.T.);
#4133=ORIENTED_EDGE('',*,*,#3119,.T.);
#4134=ORIENTED_EDGE('',*,*,#3119,.F.);
#4135=ORIENTED_EDGE('',*,*,#3120,.T.);
#4136=ORIENTED_EDGE('',*,*,#3120,.F.);
#4137=ORIENTED_EDGE('',*,*,#3121,.T.);
#4138=ORIENTED_EDGE('',*,*,#3121,.F.);
#4139=ORIENTED_EDGE('',*,*,#3122,.T.);
#4140=ORIENTED_EDGE('',*,*,#3122,.F.);
#4141=ORIENTED_EDGE('',*,*,#3123,.T.);
#4142=ORIENTED_EDGE('',*,*,#3123,.F.);
#4143=ORIENTED_EDGE('',*,*,#3124,.T.);
#4144=ORIENTED_EDGE('',*,*,#3124,.F.);
#4145=ORIENTED_EDGE('',*,*,#3125,.T.);
#4146=ORIENTED_EDGE('',*,*,#3125,.F.);
#4147=ORIENTED_EDGE('',*,*,#3126,.F.);
#4148=ORIENTED_EDGE('',*,*,#3127,.T.);
#4149=ORIENTED_EDGE('',*,*,#3128,.T.);
#4150=ORIENTED_EDGE('',*,*,#3127,.F.);
#4151=ORIENTED_EDGE('',*,*,#3129,.T.);
#4152=ORIENTED_EDGE('',*,*,#3129,.F.);
#4153=ORIENTED_EDGE('',*,*,#3130,.F.);
#4154=ORIENTED_EDGE('',*,*,#3131,.T.);
#4155=ORIENTED_EDGE('',*,*,#3126,.T.);
#4156=ORIENTED_EDGE('',*,*,#3131,.F.);
#4157=ORIENTED_EDGE('',*,*,#3128,.F.);
#4158=ORIENTED_EDGE('',*,*,#3130,.T.);
#4159=ORIENTED_EDGE('',*,*,#3132,.F.);
#4160=ORIENTED_EDGE('',*,*,#3133,.T.);
#4161=ORIENTED_EDGE('',*,*,#3134,.T.);
#4162=ORIENTED_EDGE('',*,*,#3133,.F.);
#4163=ORIENTED_EDGE('',*,*,#3135,.T.);
#4164=ORIENTED_EDGE('',*,*,#3135,.F.);
#4165=ORIENTED_EDGE('',*,*,#3136,.F.);
#4166=ORIENTED_EDGE('',*,*,#3137,.T.);
#4167=ORIENTED_EDGE('',*,*,#3132,.T.);
#4168=ORIENTED_EDGE('',*,*,#3137,.F.);
#4169=ORIENTED_EDGE('',*,*,#3134,.F.);
#4170=ORIENTED_EDGE('',*,*,#3136,.T.);
#4171=ORIENTED_EDGE('',*,*,#3138,.F.);
#4172=ORIENTED_EDGE('',*,*,#3139,.T.);
#4173=ORIENTED_EDGE('',*,*,#3140,.T.);
#4174=ORIENTED_EDGE('',*,*,#3139,.F.);
#4175=ORIENTED_EDGE('',*,*,#3141,.T.);
#4176=ORIENTED_EDGE('',*,*,#3141,.F.);
#4177=ORIENTED_EDGE('',*,*,#3142,.F.);
#4178=ORIENTED_EDGE('',*,*,#3143,.T.);
#4179=ORIENTED_EDGE('',*,*,#3138,.T.);
#4180=ORIENTED_EDGE('',*,*,#3143,.F.);
#4181=ORIENTED_EDGE('',*,*,#3140,.F.);
#4182=ORIENTED_EDGE('',*,*,#3142,.T.);
#4183=ORIENTED_EDGE('',*,*,#3144,.F.);
#4184=ORIENTED_EDGE('',*,*,#3145,.T.);
#4185=ORIENTED_EDGE('',*,*,#3146,.T.);
#4186=ORIENTED_EDGE('',*,*,#3145,.F.);
#4187=ORIENTED_EDGE('',*,*,#3147,.T.);
#4188=ORIENTED_EDGE('',*,*,#3147,.F.);
#4189=ORIENTED_EDGE('',*,*,#3148,.F.);
#4190=ORIENTED_EDGE('',*,*,#3149,.T.);
#4191=ORIENTED_EDGE('',*,*,#3144,.T.);
#4192=ORIENTED_EDGE('',*,*,#3149,.F.);
#4193=ORIENTED_EDGE('',*,*,#3146,.F.);
#4194=ORIENTED_EDGE('',*,*,#3148,.T.);
#4195=ORIENTED_EDGE('',*,*,#3150,.F.);
#4196=ORIENTED_EDGE('',*,*,#3151,.T.);
#4197=ORIENTED_EDGE('',*,*,#3152,.T.);
#4198=ORIENTED_EDGE('',*,*,#3151,.F.);
#4199=ORIENTED_EDGE('',*,*,#3153,.T.);
#4200=ORIENTED_EDGE('',*,*,#3153,.F.);
#4201=ORIENTED_EDGE('',*,*,#3154,.F.);
#4202=ORIENTED_EDGE('',*,*,#3155,.T.);
#4203=ORIENTED_EDGE('',*,*,#3150,.T.);
#4204=ORIENTED_EDGE('',*,*,#3155,.F.);
#4205=ORIENTED_EDGE('',*,*,#3152,.F.);
#4206=ORIENTED_EDGE('',*,*,#3154,.T.);
#4207=ORIENTED_EDGE('',*,*,#3156,.F.);
#4208=ORIENTED_EDGE('',*,*,#3157,.T.);
#4209=ORIENTED_EDGE('',*,*,#3158,.T.);
#4210=ORIENTED_EDGE('',*,*,#3157,.F.);
#4211=ORIENTED_EDGE('',*,*,#3159,.T.);
#4212=ORIENTED_EDGE('',*,*,#3159,.F.);
#4213=ORIENTED_EDGE('',*,*,#3160,.F.);
#4214=ORIENTED_EDGE('',*,*,#3161,.T.);
#4215=ORIENTED_EDGE('',*,*,#3156,.T.);
#4216=ORIENTED_EDGE('',*,*,#3161,.F.);
#4217=ORIENTED_EDGE('',*,*,#3158,.F.);
#4218=ORIENTED_EDGE('',*,*,#3160,.T.);
#4219=ORIENTED_EDGE('',*,*,#3162,.F.);
#4220=ORIENTED_EDGE('',*,*,#3163,.T.);
#4221=ORIENTED_EDGE('',*,*,#3164,.T.);
#4222=ORIENTED_EDGE('',*,*,#3163,.F.);
#4223=ORIENTED_EDGE('',*,*,#3165,.T.);
#4224=ORIENTED_EDGE('',*,*,#3165,.F.);
#4225=ORIENTED_EDGE('',*,*,#3166,.F.);
#4226=ORIENTED_EDGE('',*,*,#3167,.T.);
#4227=ORIENTED_EDGE('',*,*,#3162,.T.);
#4228=ORIENTED_EDGE('',*,*,#3167,.F.);
#4229=ORIENTED_EDGE('',*,*,#3164,.F.);
#4230=ORIENTED_EDGE('',*,*,#3166,.T.);
#4231=ORIENTED_EDGE('',*,*,#3168,.F.);
#4232=ORIENTED_EDGE('',*,*,#3169,.T.);
#4233=ORIENTED_EDGE('',*,*,#3170,.T.);
#4234=ORIENTED_EDGE('',*,*,#3169,.F.);
#4235=ORIENTED_EDGE('',*,*,#3171,.T.);
#4236=ORIENTED_EDGE('',*,*,#3171,.F.);
#4237=ORIENTED_EDGE('',*,*,#3172,.F.);
#4238=ORIENTED_EDGE('',*,*,#3173,.T.);
#4239=ORIENTED_EDGE('',*,*,#3168,.T.);
#4240=ORIENTED_EDGE('',*,*,#3173,.F.);
#4241=ORIENTED_EDGE('',*,*,#3170,.F.);
#4242=ORIENTED_EDGE('',*,*,#3172,.T.);
#4243=ORIENTED_EDGE('',*,*,#3174,.T.);
#4244=ORIENTED_EDGE('',*,*,#3175,.T.);
#4245=ORIENTED_EDGE('',*,*,#3176,.F.);
#4246=ORIENTED_EDGE('',*,*,#3175,.F.);
#4247=ORIENTED_EDGE('',*,*,#3177,.T.);
#4248=ORIENTED_EDGE('',*,*,#3178,.T.);
#4249=ORIENTED_EDGE('',*,*,#3179,.F.);
#4250=ORIENTED_EDGE('',*,*,#3178,.F.);
#4251=ORIENTED_EDGE('',*,*,#3179,.T.);
#4252=ORIENTED_EDGE('',*,*,#3174,.F.);
#4253=ORIENTED_EDGE('',*,*,#3177,.F.);
#4254=ORIENTED_EDGE('',*,*,#3176,.T.);
#4255=ORIENTED_EDGE('',*,*,#3180,.F.);
#4256=ORIENTED_EDGE('',*,*,#3181,.T.);
#4257=ORIENTED_EDGE('',*,*,#3182,.F.);
#4258=ORIENTED_EDGE('',*,*,#3183,.F.);
#4259=ORIENTED_EDGE('',*,*,#3181,.F.);
#4260=ORIENTED_EDGE('',*,*,#3184,.F.);
#4261=ORIENTED_EDGE('',*,*,#3185,.F.);
#4262=ORIENTED_EDGE('',*,*,#3186,.T.);
#4263=ORIENTED_EDGE('',*,*,#3187,.F.);
#4264=ORIENTED_EDGE('',*,*,#3186,.F.);
#4265=ORIENTED_EDGE('',*,*,#3184,.T.);
#4266=ORIENTED_EDGE('',*,*,#3185,.T.);
#4267=ORIENTED_EDGE('',*,*,#3188,.T.);
#4268=ORIENTED_EDGE('',*,*,#3189,.T.);
#4269=ORIENTED_EDGE('',*,*,#3190,.T.);
#4270=ORIENTED_EDGE('',*,*,#3188,.F.);
#4271=ORIENTED_EDGE('',*,*,#3191,.T.);
#4272=ORIENTED_EDGE('',*,*,#3192,.T.);
#4273=ORIENTED_EDGE('',*,*,#3189,.F.);
#4274=ORIENTED_EDGE('',*,*,#3190,.F.);
#4275=ORIENTED_EDGE('',*,*,#3192,.F.);
#4276=ORIENTED_EDGE('',*,*,#3193,.F.);
#4277=ORIENTED_EDGE('',*,*,#3194,.T.);
#4278=ORIENTED_EDGE('',*,*,#3195,.T.);
#4279=ORIENTED_EDGE('',*,*,#3194,.F.);
#4280=ORIENTED_EDGE('',*,*,#3195,.F.);
#4281=ORIENTED_EDGE('',*,*,#3196,.T.);
#4282=ORIENTED_EDGE('',*,*,#3182,.T.);
#4283=ORIENTED_EDGE('',*,*,#3183,.T.);
#4284=ORIENTED_EDGE('',*,*,#3196,.F.);
#4285=ORIENTED_EDGE('',*,*,#3187,.T.);
#4286=ORIENTED_EDGE('',*,*,#3180,.T.);
#4287=ORIENTED_EDGE('',*,*,#3191,.F.);
#4288=ORIENTED_EDGE('',*,*,#3193,.T.);
#4289=ORIENTED_EDGE('',*,*,#3197,.F.);
#4290=ORIENTED_EDGE('',*,*,#3198,.T.);
#4291=ORIENTED_EDGE('',*,*,#3199,.F.);
#4292=ORIENTED_EDGE('',*,*,#3198,.F.);
#4293=ORIENTED_EDGE('',*,*,#3200,.F.);
#4294=ORIENTED_EDGE('',*,*,#3201,.T.);
#4295=ORIENTED_EDGE('',*,*,#3202,.F.);
#4296=ORIENTED_EDGE('',*,*,#3201,.F.);
#4297=ORIENTED_EDGE('',*,*,#3202,.T.);
#4298=ORIENTED_EDGE('',*,*,#3203,.T.);
#4299=ORIENTED_EDGE('',*,*,#3204,.T.);
#4300=ORIENTED_EDGE('',*,*,#3205,.T.);
#4301=ORIENTED_EDGE('',*,*,#3203,.F.);
#4302=ORIENTED_EDGE('',*,*,#3206,.T.);
#4303=ORIENTED_EDGE('',*,*,#3207,.T.);
#4304=ORIENTED_EDGE('',*,*,#3204,.F.);
#4305=ORIENTED_EDGE('',*,*,#3205,.F.);
#4306=ORIENTED_EDGE('',*,*,#3207,.F.);
#4307=ORIENTED_EDGE('',*,*,#3208,.F.);
#4308=ORIENTED_EDGE('',*,*,#3209,.T.);
#4309=ORIENTED_EDGE('',*,*,#3210,.T.);
#4310=ORIENTED_EDGE('',*,*,#3209,.F.);
#4311=ORIENTED_EDGE('',*,*,#3210,.F.);
#4312=ORIENTED_EDGE('',*,*,#3211,.T.);
#4313=ORIENTED_EDGE('',*,*,#3197,.T.);
#4314=ORIENTED_EDGE('',*,*,#3211,.F.);
#4315=ORIENTED_EDGE('',*,*,#3208,.T.);
#4316=ORIENTED_EDGE('',*,*,#3206,.F.);
#4317=ORIENTED_EDGE('',*,*,#3199,.T.);
#4318=ORIENTED_EDGE('',*,*,#3200,.T.);
#4610=CYLINDRICAL_SURFACE('',#5584,7.5);
#4611=CYLINDRICAL_SURFACE('',#5589,11.);
#4612=CYLINDRICAL_SURFACE('',#5591,11.);
#4613=CYLINDRICAL_SURFACE('',#5600,14.);
#4614=CYLINDRICAL_SURFACE('',#5606,14.);
#4615=CYLINDRICAL_SURFACE('',#5612,17.5);
#4616=CYLINDRICAL_SURFACE('',#5709,12.5);
#4617=CYLINDRICAL_SURFACE('',#5712,13.25);
#4618=CYLINDRICAL_SURFACE('',#5727,13.775);
#4619=CYLINDRICAL_SURFACE('',#5735,11.225);
#4620=CYLINDRICAL_SURFACE('',#5746,11.225);
#4621=CYLINDRICAL_SURFACE('',#5754,13.775);
#4852=ADVANCED_FACE('',(#841),#131,.F.);
#4853=ADVANCED_FACE('',(#842),#116,.F.);
#4854=ADVANCED_FACE('',(#843),#4610,.F.);
#4855=ADVANCED_FACE('',(#844),#117,.F.);
#4856=ADVANCED_FACE('',(#845),#4611,.T.);
#4857=ADVANCED_FACE('',(#846),#4612,.T.);
#4858=ADVANCED_FACE('',(#847,#418),#570,.F.);
#4859=ADVANCED_FACE('',(#848,#419),#571,.F.);
#4860=ADVANCED_FACE('',(#849),#317,.T.);
#4861=ADVANCED_FACE('',(#850),#118,.T.);
#4862=ADVANCED_FACE('',(#851),#4613,.F.);
#4863=ADVANCED_FACE('',(#852),#132,.F.);
#4864=ADVANCED_FACE('',(#853),#4614,.F.);
#4865=ADVANCED_FACE('',(#854),#119,.T.);
#4866=ADVANCED_FACE('',(#855),#4615,.T.);
#4867=ADVANCED_FACE('',(#856,#420),#572,.F.);
#4868=ADVANCED_FACE('',(#857,#421),#573,.F.);
#4869=ADVANCED_FACE('',(#858),#318,.T.);
#4870=ADVANCED_FACE('',(#859),#319,.T.);
#4871=ADVANCED_FACE('',(#860),#320,.T.);
#4872=ADVANCED_FACE('',(#861),#321,.T.);
#4873=ADVANCED_FACE('',(#862),#322,.T.);
#4874=ADVANCED_FACE('',(#863),#323,.T.);
#4875=ADVANCED_FACE('',(#864),#324,.T.);
#4876=ADVANCED_FACE('',(#865),#133,.T.);
#4877=ADVANCED_FACE('',(#866,#422,#423),#325,.F.);
#4878=ADVANCED_FACE('',(#867,#424),#574,.T.);
#4879=ADVANCED_FACE('',(#868,#425),#575,.T.);
#4880=ADVANCED_FACE('',(#869),#134,.T.);
#4881=ADVANCED_FACE('',(#870,#426,#427),#326,.F.);
#4882=ADVANCED_FACE('',(#871,#428),#576,.T.);
#4883=ADVANCED_FACE('',(#872,#429),#577,.T.);
#4884=ADVANCED_FACE('',(#873),#135,.T.);
#4885=ADVANCED_FACE('',(#874,#430,#431),#327,.F.);
#4886=ADVANCED_FACE('',(#875,#432),#578,.T.);
#4887=ADVANCED_FACE('',(#876,#433),#579,.T.);
#4888=ADVANCED_FACE('',(#877),#136,.T.);
#4889=ADVANCED_FACE('',(#878,#434,#435),#328,.F.);
#4890=ADVANCED_FACE('',(#879,#436),#580,.T.);
#4891=ADVANCED_FACE('',(#880,#437),#581,.T.);
#4892=ADVANCED_FACE('',(#881),#137,.T.);
#4893=ADVANCED_FACE('',(#882,#438,#439),#329,.F.);
#4894=ADVANCED_FACE('',(#883,#440),#582,.T.);
#4895=ADVANCED_FACE('',(#884,#441),#583,.T.);
#4896=ADVANCED_FACE('',(#885),#138,.T.);
#4897=ADVANCED_FACE('',(#886,#442,#443),#330,.F.);
#4898=ADVANCED_FACE('',(#887,#444),#584,.T.);
#4899=ADVANCED_FACE('',(#888,#445),#585,.T.);
#4900=ADVANCED_FACE('',(#889),#139,.T.);
#4901=ADVANCED_FACE('',(#890,#446,#447),#331,.F.);
#4902=ADVANCED_FACE('',(#891,#448),#586,.T.);
#4903=ADVANCED_FACE('',(#892,#449),#587,.T.);
#4904=ADVANCED_FACE('',(#893),#140,.T.);
#4905=ADVANCED_FACE('',(#894,#450,#451),#332,.F.);
#4906=ADVANCED_FACE('',(#895,#452),#588,.T.);
#4907=ADVANCED_FACE('',(#896,#453),#589,.T.);
#4908=ADVANCED_FACE('',(#897),#4616,.F.);
#4909=ADVANCED_FACE('',(#898),#4617,.T.);
#4910=ADVANCED_FACE('',(#899,#454),#590,.T.);
#4911=ADVANCED_FACE('',(#900,#455),#591,.F.);
#4912=ADVANCED_FACE('',(#901),#141,.T.);
#4913=ADVANCED_FACE('',(#902),#142,.T.);
#4914=ADVANCED_FACE('',(#903),#4618,.T.);
#4915=ADVANCED_FACE('',(#904),#120,.T.);
#4916=ADVANCED_FACE('',(#905),#121,.F.);
#4917=ADVANCED_FACE('',(#906),#4619,.F.);
#4918=ADVANCED_FACE('',(#907,#456),#592,.F.);
#4919=ADVANCED_FACE('',(#908,#457),#593,.F.);
#4920=ADVANCED_FACE('',(#909),#143,.T.);
#4921=ADVANCED_FACE('',(#910),#144,.T.);
#4922=ADVANCED_FACE('',(#911),#4620,.F.);
#4923=ADVANCED_FACE('',(#912),#122,.F.);
#4924=ADVANCED_FACE('',(#913),#123,.T.);
#4925=ADVANCED_FACE('',(#914),#4621,.T.);
#4926=ADVANCED_FACE('',(#915,#458),#594,.F.);
#4927=ADVANCED_FACE('',(#916,#459),#595,.F.);
#5000=CLOSED_SHELL('',(#4852,#4853,#4854,#4855,#4856,#4857,#4858,#4859));
#5001=CLOSED_SHELL('',(#4860));
#5002=CLOSED_SHELL('',(#4861,#4862,#4863,#4864,#4865,#4866,#4867,#4868));
#5003=CLOSED_SHELL('',(#4869));
#5004=CLOSED_SHELL('',(#4870));
#5005=CLOSED_SHELL('',(#4871));
#5006=CLOSED_SHELL('',(#4872));
#5007=CLOSED_SHELL('',(#4873));
#5008=CLOSED_SHELL('',(#4874));
#5009=CLOSED_SHELL('',(#4875));
#5010=CLOSED_SHELL('',(#4876,#4877,#4878,#4879));
#5011=CLOSED_SHELL('',(#4880,#4881,#4882,#4883));
#5012=CLOSED_SHELL('',(#4884,#4885,#4886,#4887));
#5013=CLOSED_SHELL('',(#4888,#4889,#4890,#4891));
#5014=CLOSED_SHELL('',(#4892,#4893,#4894,#4895));
#5015=CLOSED_SHELL('',(#4896,#4897,#4898,#4899));
#5016=CLOSED_SHELL('',(#4900,#4901,#4902,#4903));
#5017=CLOSED_SHELL('',(#4904,#4905,#4906,#4907));
#5018=CLOSED_SHELL('',(#4908,#4909,#4910,#4911));
#5019=CLOSED_SHELL('',(#4912,#4913,#4914,#4915,#4916,#4917,#4918,#4919));
#5020=CLOSED_SHELL('',(#4920,#4921,#4922,#4923,#4924,#4925,#4926,#4927));
#5576=AXIS2_PLACEMENT_3D('',#8650,#6868,#6869);
#5577=AXIS2_PLACEMENT_3D('',#8651,#6870,#6871);
#5578=AXIS2_PLACEMENT_3D('',#8653,#6872,#6873);
#5579=AXIS2_PLACEMENT_3D('',#8655,#6874,#6875);
#5580=AXIS2_PLACEMENT_3D('',#8656,#6876,#6877);
#5581=AXIS2_PLACEMENT_3D('',#8657,#6878,#6879);
#5582=AXIS2_PLACEMENT_3D('',#8659,#6880,#6881);
#5583=AXIS2_PLACEMENT_3D('',#8662,#6883,#6884);
#5584=AXIS2_PLACEMENT_3D('',#8663,#6885,#6886);
#5585=AXIS2_PLACEMENT_3D('',#8666,#6887,#6888);
#5586=AXIS2_PLACEMENT_3D('',#8667,#6889,#6890);
#5587=AXIS2_PLACEMENT_3D('',#8669,#6892,#6893);
#5588=AXIS2_PLACEMENT_3D('',#8672,#6895,#6896);
#5589=AXIS2_PLACEMENT_3D('',#8673,#6897,#6898);
#5590=AXIS2_PLACEMENT_3D('',#8676,#6900,#6901);
#5591=AXIS2_PLACEMENT_3D('',#8677,#6902,#6903);
#5592=AXIS2_PLACEMENT_3D('',#8679,#6904,#6905);
#5593=AXIS2_PLACEMENT_3D('',#8681,#6907,#6908);
#5594=AXIS2_PLACEMENT_3D('',#8682,#6909,#6910);
#5595=AXIS2_PLACEMENT_3D('',#8683,#6911,#6912);
#5596=AXIS2_PLACEMENT_3D('',#8686,#6913,#6914);
#5597=AXIS2_PLACEMENT_3D('',#8687,#6915,#6916);
#5598=AXIS2_PLACEMENT_3D('',#8689,#6917,#6918);
#5599=AXIS2_PLACEMENT_3D('',#8692,#6920,#6921);
#5600=AXIS2_PLACEMENT_3D('',#8693,#6922,#6923);
#5601=AXIS2_PLACEMENT_3D('',#8695,#6924,#6925);
#5602=AXIS2_PLACEMENT_3D('',#8698,#6927,#6928);
#5603=AXIS2_PLACEMENT_3D('',#8699,#6929,#6930);
#5604=AXIS2_PLACEMENT_3D('',#8701,#6931,#6932);
#5605=AXIS2_PLACEMENT_3D('',#8702,#6933,#6934);
#5606=AXIS2_PLACEMENT_3D('',#8703,#6935,#6936);
#5607=AXIS2_PLACEMENT_3D('',#8706,#6938,#6939);
#5608=AXIS2_PLACEMENT_3D('',#8707,#6940,#6941);
#5609=AXIS2_PLACEMENT_3D('',#8710,#6942,#6943);
#5610=AXIS2_PLACEMENT_3D('',#8713,#6945,#6946);
#5611=AXIS2_PLACEMENT_3D('',#8714,#6947,#6948);
#5612=AXIS2_PLACEMENT_3D('',#8715,#6949,#6950);
#5613=AXIS2_PLACEMENT_3D('',#8717,#6952,#6953);
#5614=AXIS2_PLACEMENT_3D('',#8718,#6954,#6955);
#5615=AXIS2_PLACEMENT_3D('',#8719,#6956,#6957);
#5616=AXIS2_PLACEMENT_3D('',#8722,#6958,#6959);
#5617=AXIS2_PLACEMENT_3D('',#8723,#6960,#6961);
#5618=AXIS2_PLACEMENT_3D('',#8726,#6962,#6963);
#5619=AXIS2_PLACEMENT_3D('',#8727,#6964,#6965);
#5620=AXIS2_PLACEMENT_3D('',#8730,#6966,#6967);
#5621=AXIS2_PLACEMENT_3D('',#8731,#6968,#6969);
#5622=AXIS2_PLACEMENT_3D('',#8734,#6970,#6971);
#5623=AXIS2_PLACEMENT_3D('',#8735,#6972,#6973);
#5624=AXIS2_PLACEMENT_3D('',#8738,#6974,#6975);
#5625=AXIS2_PLACEMENT_3D('',#8739,#6976,#6977);
#5626=AXIS2_PLACEMENT_3D('',#8742,#6978,#6979);
#5627=AXIS2_PLACEMENT_3D('',#8743,#6980,#6981);
#5628=AXIS2_PLACEMENT_3D('',#8746,#6982,#6983);
#5629=AXIS2_PLACEMENT_3D('',#8747,#6984,#6985);
#5630=AXIS2_PLACEMENT_3D('',#8749,#6986,#6987);
#5631=AXIS2_PLACEMENT_3D('',#8751,#6988,#6989);
#5632=AXIS2_PLACEMENT_3D('',#8752,#6990,#6991);
#5633=AXIS2_PLACEMENT_3D('',#8753,#6992,#6993);
#5634=AXIS2_PLACEMENT_3D('',#8756,#6994,#6995);
#5635=AXIS2_PLACEMENT_3D('',#8758,#6996,#6997);
#5636=AXIS2_PLACEMENT_3D('',#8760,#6998,#6999);
#5637=AXIS2_PLACEMENT_3D('',#8761,#7000,#7001);
#5638=AXIS2_PLACEMENT_3D('',#8762,#7002,#7003);
#5639=AXIS2_PLACEMENT_3D('',#8763,#7004,#7005);
#5640=AXIS2_PLACEMENT_3D('',#8765,#7006,#7007);
#5641=AXIS2_PLACEMENT_3D('',#8767,#7008,#7009);
#5642=AXIS2_PLACEMENT_3D('',#8768,#7010,#7011);
#5643=AXIS2_PLACEMENT_3D('',#8769,#7012,#7013);
#5644=AXIS2_PLACEMENT_3D('',#8772,#7014,#7015);
#5645=AXIS2_PLACEMENT_3D('',#8774,#7016,#7017);
#5646=AXIS2_PLACEMENT_3D('',#8776,#7018,#7019);
#5647=AXIS2_PLACEMENT_3D('',#8777,#7020,#7021);
#5648=AXIS2_PLACEMENT_3D('',#8778,#7022,#7023);
#5649=AXIS2_PLACEMENT_3D('',#8779,#7024,#7025);
#5650=AXIS2_PLACEMENT_3D('',#8781,#7026,#7027);
#5651=AXIS2_PLACEMENT_3D('',#8783,#7028,#7029);
#5652=AXIS2_PLACEMENT_3D('',#8784,#7030,#7031);
#5653=AXIS2_PLACEMENT_3D('',#8785,#7032,#7033);
#5654=AXIS2_PLACEMENT_3D('',#8788,#7034,#7035);
#5655=AXIS2_PLACEMENT_3D('',#8790,#7036,#7037);
#5656=AXIS2_PLACEMENT_3D('',#8792,#7038,#7039);
#5657=AXIS2_PLACEMENT_3D('',#8793,#7040,#7041);
#5658=AXIS2_PLACEMENT_3D('',#8794,#7042,#7043);
#5659=AXIS2_PLACEMENT_3D('',#8795,#7044,#7045);
#5660=AXIS2_PLACEMENT_3D('',#8797,#7046,#7047);
#5661=AXIS2_PLACEMENT_3D('',#8799,#7048,#7049);
#5662=AXIS2_PLACEMENT_3D('',#8800,#7050,#7051);
#5663=AXIS2_PLACEMENT_3D('',#8801,#7052,#7053);
#5664=AXIS2_PLACEMENT_3D('',#8804,#7054,#7055);
#5665=AXIS2_PLACEMENT_3D('',#8806,#7056,#7057);
#5666=AXIS2_PLACEMENT_3D('',#8808,#7058,#7059);
#5667=AXIS2_PLACEMENT_3D('',#8809,#7060,#7061);
#5668=AXIS2_PLACEMENT_3D('',#8810,#7062,#7063);
#5669=AXIS2_PLACEMENT_3D('',#8811,#7064,#7065);
#5670=AXIS2_PLACEMENT_3D('',#8813,#7066,#7067);
#5671=AXIS2_PLACEMENT_3D('',#8815,#7068,#7069);
#5672=AXIS2_PLACEMENT_3D('',#8816,#7070,#7071);
#5673=AXIS2_PLACEMENT_3D('',#8817,#7072,#7073);
#5674=AXIS2_PLACEMENT_3D('',#8820,#7074,#7075);
#5675=AXIS2_PLACEMENT_3D('',#8822,#7076,#7077);
#5676=AXIS2_PLACEMENT_3D('',#8824,#7078,#7079);
#5677=AXIS2_PLACEMENT_3D('',#8825,#7080,#7081);
#5678=AXIS2_PLACEMENT_3D('',#8826,#7082,#7083);
#5679=AXIS2_PLACEMENT_3D('',#8827,#7084,#7085);
#5680=AXIS2_PLACEMENT_3D('',#8829,#7086,#7087);
#5681=AXIS2_PLACEMENT_3D('',#8831,#7088,#7089);
#5682=AXIS2_PLACEMENT_3D('',#8832,#7090,#7091);
#5683=AXIS2_PLACEMENT_3D('',#8833,#7092,#7093);
#5684=AXIS2_PLACEMENT_3D('',#8836,#7094,#7095);
#5685=AXIS2_PLACEMENT_3D('',#8838,#7096,#7097);
#5686=AXIS2_PLACEMENT_3D('',#8840,#7098,#7099);
#5687=AXIS2_PLACEMENT_3D('',#8841,#7100,#7101);
#5688=AXIS2_PLACEMENT_3D('',#8842,#7102,#7103);
#5689=AXIS2_PLACEMENT_3D('',#8843,#7104,#7105);
#5690=AXIS2_PLACEMENT_3D('',#8845,#7106,#7107);
#5691=AXIS2_PLACEMENT_3D('',#8847,#7108,#7109);
#5692=AXIS2_PLACEMENT_3D('',#8848,#7110,#7111);
#5693=AXIS2_PLACEMENT_3D('',#8849,#7112,#7113);
#5694=AXIS2_PLACEMENT_3D('',#8852,#7114,#7115);
#5695=AXIS2_PLACEMENT_3D('',#8854,#7116,#7117);
#5696=AXIS2_PLACEMENT_3D('',#8856,#7118,#7119);
#5697=AXIS2_PLACEMENT_3D('',#8857,#7120,#7121);
#5698=AXIS2_PLACEMENT_3D('',#8858,#7122,#7123);
#5699=AXIS2_PLACEMENT_3D('',#8859,#7124,#7125);
#5700=AXIS2_PLACEMENT_3D('',#8861,#7126,#7127);
#5701=AXIS2_PLACEMENT_3D('',#8863,#7128,#7129);
#5702=AXIS2_PLACEMENT_3D('',#8864,#7130,#7131);
#5703=AXIS2_PLACEMENT_3D('',#8865,#7132,#7133);
#5704=AXIS2_PLACEMENT_3D('',#8868,#7134,#7135);
#5705=AXIS2_PLACEMENT_3D('',#8870,#7136,#7137);
#5706=AXIS2_PLACEMENT_3D('',#8872,#7138,#7139);
#5707=AXIS2_PLACEMENT_3D('',#8873,#7140,#7141);
#5708=AXIS2_PLACEMENT_3D('',#8874,#7142,#7143);
#5709=AXIS2_PLACEMENT_3D('',#8875,#7144,#7145);
#5710=AXIS2_PLACEMENT_3D('',#8877,#7146,#7147);
#5711=AXIS2_PLACEMENT_3D('',#8880,#7149,#7150);
#5712=AXIS2_PLACEMENT_3D('',#8881,#7151,#7152);
#5713=AXIS2_PLACEMENT_3D('',#8883,#7153,#7154);
#5714=AXIS2_PLACEMENT_3D('',#8886,#7156,#7157);
#5715=AXIS2_PLACEMENT_3D('',#8887,#7158,#7159);
#5716=AXIS2_PLACEMENT_3D('',#8888,#7160,#7161);
#5717=AXIS2_PLACEMENT_3D('',#8889,#7162,#7163);
#5718=AXIS2_PLACEMENT_3D('',#8891,#7164,#7165);
#5719=AXIS2_PLACEMENT_3D('',#8893,#7166,#7167);
#5720=AXIS2_PLACEMENT_3D('',#8895,#7168,#7169);
#5721=AXIS2_PLACEMENT_3D('',#8896,#7170,#7171);
#5722=AXIS2_PLACEMENT_3D('',#8897,#7172,#7173);
#5723=AXIS2_PLACEMENT_3D('',#8900,#7174,#7175);
#5724=AXIS2_PLACEMENT_3D('',#8901,#7176,#7177);
#5725=AXIS2_PLACEMENT_3D('',#8903,#7178,#7179);
#5726=AXIS2_PLACEMENT_3D('',#8904,#7180,#7181);
#5727=AXIS2_PLACEMENT_3D('',#8905,#7182,#7183);
#5728=AXIS2_PLACEMENT_3D('',#8909,#7185,#7186);
#5729=AXIS2_PLACEMENT_3D('',#8910,#7187,#7188);
#5730=AXIS2_PLACEMENT_3D('',#8911,#7189,#7190);
#5731=AXIS2_PLACEMENT_3D('',#8913,#7191,#7192);
#5732=AXIS2_PLACEMENT_3D('',#8915,#7194,#7195);
#5733=AXIS2_PLACEMENT_3D('',#8917,#7196,#7197);
#5734=AXIS2_PLACEMENT_3D('',#8920,#7199,#7200);
#5735=AXIS2_PLACEMENT_3D('',#8921,#7201,#7202);
#5736=AXIS2_PLACEMENT_3D('',#8923,#7204,#7205);
#5737=AXIS2_PLACEMENT_3D('',#8924,#7206,#7207);
#5738=AXIS2_PLACEMENT_3D('',#8925,#7208,#7209);
#5739=AXIS2_PLACEMENT_3D('',#8927,#7210,#7211);
#5740=AXIS2_PLACEMENT_3D('',#8929,#7212,#7213);
#5741=AXIS2_PLACEMENT_3D('',#8930,#7214,#7215);
#5742=AXIS2_PLACEMENT_3D('',#8931,#7216,#7217);
#5743=AXIS2_PLACEMENT_3D('',#8933,#7218,#7219);
#5744=AXIS2_PLACEMENT_3D('',#8935,#7220,#7221);
#5745=AXIS2_PLACEMENT_3D('',#8936,#7222,#7223);
#5746=AXIS2_PLACEMENT_3D('',#8937,#7224,#7225);
#5747=AXIS2_PLACEMENT_3D('',#8941,#7227,#7228);
#5748=AXIS2_PLACEMENT_3D('',#8942,#7229,#7230);
#5749=AXIS2_PLACEMENT_3D('',#8943,#7231,#7232);
#5750=AXIS2_PLACEMENT_3D('',#8945,#7233,#7234);
#5751=AXIS2_PLACEMENT_3D('',#8947,#7236,#7237);
#5752=AXIS2_PLACEMENT_3D('',#8949,#7238,#7239);
#5753=AXIS2_PLACEMENT_3D('',#8952,#7241,#7242);
#5754=AXIS2_PLACEMENT_3D('',#8953,#7243,#7244);
#5755=AXIS2_PLACEMENT_3D('',#8955,#7246,#7247);
#5756=AXIS2_PLACEMENT_3D('',#8956,#7248,#7249);
#6868=DIRECTION('axis',(0.,0.,1.));
#6869=DIRECTION('refdir',(1.,0.,0.));
#6870=DIRECTION('center_axis',(0.,-1.83697019872103E-16,1.));
#6871=DIRECTION('ref_axis',(0.,-1.,-1.83697019872103E-16));
#6872=DIRECTION('center_axis',(0.,-1.83697019872103E-16,1.));
#6873=DIRECTION('ref_axis',(0.,-1.,-1.83697019872103E-16));
#6874=DIRECTION('center_axis',(1.,1.22464679914735E-16,2.24963967399279E-32));
#6875=DIRECTION('ref_axis',(-1.22464679914735E-16,1.,1.83697019872103E-16));
#6876=DIRECTION('center_axis',(0.,-1.83697019872103E-16,1.));
#6877=DIRECTION('ref_axis',(0.,-1.,-1.83697019872103E-16));
#6878=DIRECTION('center_axis',(0.,-1.83697019872103E-16,1.));
#6879=DIRECTION('ref_axis',(0.,-1.,-1.83697019872103E-16));
#6880=DIRECTION('center_axis',(0.,-1.83697019872103E-16,1.));
#6881=DIRECTION('ref_axis',(0.,-1.,-1.83697019872103E-16));
#6882=DIRECTION('',(-8.65956056235486E-17,0.707106781186541,0.707106781186554));
#6883=DIRECTION('center_axis',(0.,-1.83697019872103E-16,1.));
#6884=DIRECTION('ref_axis',(0.,-1.,-1.83697019872103E-16));
#6885=DIRECTION('center_axis',(0.,-1.83697019872103E-16,1.));
#6886=DIRECTION('ref_axis',(0.,-1.,-1.83697019872103E-16));
#6887=DIRECTION('center_axis',(0.,-1.83697019872103E-16,1.));
#6888=DIRECTION('ref_axis',(0.,-1.,-1.83697019872103E-16));
#6889=DIRECTION('center_axis',(0.,-1.83697019872103E-16,1.));
#6890=DIRECTION('ref_axis',(0.,-1.,-1.83697019872103E-16));
#6891=DIRECTION('',(0.,-1.83697019872103E-16,1.));
#6892=DIRECTION('center_axis',(0.,1.83697019872103E-16,-1.));
#6893=DIRECTION('ref_axis',(0.,1.,1.83697019872103E-16));
#6894=DIRECTION('',(-8.65956056235486E-17,-0.707106781186541,-0.707106781186554));
#6895=DIRECTION('center_axis',(0.,-1.83697019872103E-16,1.));
#6896=DIRECTION('ref_axis',(0.,-1.,-1.83697019872103E-16));
#6897=DIRECTION('center_axis',(0.,-1.83697019872103E-16,1.));
#6898=DIRECTION('ref_axis',(0.,-1.,-1.83697019872103E-16));
#6899=DIRECTION('',(0.,1.83697019872103E-16,-1.));
#6900=DIRECTION('center_axis',(0.,-1.83697019872103E-16,1.));
#6901=DIRECTION('ref_axis',(0.,-1.,-1.83697019872103E-16));
#6902=DIRECTION('center_axis',(0.,-1.83697019872103E-16,1.));
#6903=DIRECTION('ref_axis',(0.,-1.,-1.83697019872103E-16));
#6904=DIRECTION('center_axis',(0.,-1.83697019872103E-16,1.));
#6905=DIRECTION('ref_axis',(0.,-1.,-1.83697019872103E-16));
#6906=DIRECTION('',(0.,1.83697019872103E-16,-1.));
#6907=DIRECTION('center_axis',(0.,1.83697019872103E-16,-1.));
#6908=DIRECTION('ref_axis',(0.,1.,1.83697019872103E-16));
#6909=DIRECTION('center_axis',(0.,-1.83697019872103E-16,1.));
#6910=DIRECTION('ref_axis',(0.,-1.,-1.83697019872103E-16));
#6911=DIRECTION('center_axis',(-1.,0.,0.));
#6912=DIRECTION('ref_axis',(0.,1.,0.));
#6913=DIRECTION('center_axis',(0.,1.22464679914735E-16,1.));
#6914=DIRECTION('ref_axis',(0.,-1.,1.22464679914735E-16));
#6915=DIRECTION('center_axis',(0.,-1.83697019872103E-16,1.));
#6916=DIRECTION('ref_axis',(0.,-1.,-1.83697019872103E-16));
#6917=DIRECTION('center_axis',(0.,-1.83697019872103E-16,1.));
#6918=DIRECTION('ref_axis',(0.,-1.,-1.83697019872103E-16));
#6919=DIRECTION('',(8.65956056235492E-17,-0.707106781186546,-0.707106781186549));
#6920=DIRECTION('center_axis',(0.,-1.83697019872103E-16,1.));
#6921=DIRECTION('ref_axis',(0.,-1.,-1.83697019872103E-16));
#6922=DIRECTION('center_axis',(0.,-1.83697019872103E-16,1.));
#6923=DIRECTION('ref_axis',(0.,-1.,-1.83697019872103E-16));
#6924=DIRECTION('center_axis',(0.,-1.83697019872103E-16,1.));
#6925=DIRECTION('ref_axis',(0.,-1.,-1.83697019872103E-16));
#6926=DIRECTION('',(0.,-1.83697019872103E-16,1.));
#6927=DIRECTION('center_axis',(0.,-1.83697019872103E-16,1.));
#6928=DIRECTION('ref_axis',(0.,-1.,-1.83697019872103E-16));
#6929=DIRECTION('center_axis',(0.,-1.83697019872103E-16,1.));
#6930=DIRECTION('ref_axis',(0.,-1.,-1.83697019872103E-16));
#6931=DIRECTION('center_axis',(1.,1.22464679914735E-16,2.24963967399279E-32));
#6932=DIRECTION('ref_axis',(-1.22464679914735E-16,1.,1.83697019872103E-16));
#6933=DIRECTION('center_axis',(0.,-1.83697019872103E-16,1.));
#6934=DIRECTION('ref_axis',(0.,-1.,-1.83697019872103E-16));
#6935=DIRECTION('center_axis',(0.,-1.83697019872103E-16,1.));
#6936=DIRECTION('ref_axis',(0.,-1.,-1.83697019872103E-16));
#6937=DIRECTION('',(0.,-1.83697019872103E-16,1.));
#6938=DIRECTION('center_axis',(0.,-1.83697019872103E-16,1.));
#6939=DIRECTION('ref_axis',(0.,-1.,-1.83697019872103E-16));
#6940=DIRECTION('center_axis',(0.,1.83697019872103E-16,-1.));
#6941=DIRECTION('ref_axis',(0.,1.,1.83697019872103E-16));
#6942=DIRECTION('center_axis',(0.,-1.83697019872103E-16,1.));
#6943=DIRECTION('ref_axis',(0.,-1.,-1.83697019872103E-16));
#6944=DIRECTION('',(8.65956056235491E-17,0.707106781186546,0.707106781186549));
#6945=DIRECTION('center_axis',(0.,-1.83697019872103E-16,1.));
#6946=DIRECTION('ref_axis',(0.,-1.,-1.83697019872103E-16));
#6947=DIRECTION('center_axis',(0.,-1.83697019872103E-16,1.));
#6948=DIRECTION('ref_axis',(0.,-1.,-1.83697019872103E-16));
#6949=DIRECTION('center_axis',(0.,-1.83697019872103E-16,1.));
#6950=DIRECTION('ref_axis',(0.,-1.,-1.83697019872103E-16));
#6951=DIRECTION('',(0.,1.83697019872103E-16,-1.));
#6952=DIRECTION('center_axis',(0.,1.83697019872103E-16,-1.));
#6953=DIRECTION('ref_axis',(0.,1.,1.83697019872103E-16));
#6954=DIRECTION('center_axis',(0.,-1.83697019872103E-16,1.));
#6955=DIRECTION('ref_axis',(0.,-1.,-1.83697019872103E-16));
#6956=DIRECTION('center_axis',(-0.707106781186546,0.707106781186549,1.29893408435324E-16));
#6957=DIRECTION('ref_axis',(0.707106781186549,0.707106781186546,-5.38036114367792E-17));
#6958=DIRECTION('center_axis',(2.16489014058874E-16,3.279199418677E-17,
1.));
#6959=DIRECTION('ref_axis',(-0.707106781186549,-0.707106781186546,1.76268291351515E-16));
#6960=DIRECTION('center_axis',(3.71625375700965E-15,1.,1.83697019872103E-16));
#6961=DIRECTION('ref_axis',(1.,-3.71625375700965E-15,-1.83697019872104E-16));
#6962=DIRECTION('center_axis',(3.06161699786839E-16,-1.83697019872104E-16,
1.));
#6963=DIRECTION('ref_axis',(-1.,3.71625375700965E-15,3.06161699786839E-16));
#6964=DIRECTION('center_axis',(0.707106781186551,0.707106781186544,1.29893408435323E-16));
#6965=DIRECTION('ref_axis',(0.707106781186544,-0.707106781186551,-3.13590428307427E-16));
#6966=DIRECTION('center_axis',(2.16489014058872E-16,-4.00186033930977E-16,
1.));
#6967=DIRECTION('ref_axis',(-0.707106781186544,0.707106781186551,4.36055108222162E-16));
#6968=DIRECTION('center_axis',(1.,0.,0.));
#6969=DIRECTION('ref_axis',(0.,-1.,-3.67394039744206E-16));
#6970=DIRECTION('center_axis',(0.,-4.89858719658941E-16,1.));
#6971=DIRECTION('ref_axis',(0.,1.,4.89858719658941E-16));
#6972=DIRECTION('center_axis',(0.707106781186541,-0.707106781186554,-1.29893408435325E-16));
#6973=DIRECTION('ref_axis',(-0.707106781186554,-0.707106781186541,-3.13590428307426E-16));
#6974=DIRECTION('center_axis',(-2.16489014058876E-16,-4.00186033930974E-16,
1.));
#6975=DIRECTION('ref_axis',(0.707106781186554,0.707106781186541,4.36055108222162E-16));
#6976=DIRECTION('center_axis',(-1.05293856448607E-14,-1.,-1.83697019872103E-16));
#6977=DIRECTION('ref_axis',(-1.,1.05293856448607E-14,-1.83697019872101E-16));
#6978=DIRECTION('center_axis',(-3.06161699786838E-16,-1.836970198721E-16,
1.));
#6979=DIRECTION('ref_axis',(1.,-1.05293856448607E-14,3.06161699786836E-16));
#6980=DIRECTION('center_axis',(-0.707106781186556,-0.707106781186539,-1.29893408435322E-16));
#6981=DIRECTION('ref_axis',(-0.707106781186539,0.707106781186556,-5.38036114367774E-17));
#6982=DIRECTION('center_axis',(-2.1648901405887E-16,3.27919941867732E-17,
1.));
#6983=DIRECTION('ref_axis',(0.707106781186539,-0.707106781186556,1.76268291351513E-16));
#6984=DIRECTION('center_axis',(0.,1.,0.));
#6985=DIRECTION('ref_axis',(0.,0.,1.));
#6986=DIRECTION('center_axis',(0.,1.,0.));
#6987=DIRECTION('ref_axis',(0.,0.,1.));
#6988=DIRECTION('center_axis',(-1.,0.,1.22464679914735E-16));
#6989=DIRECTION('ref_axis',(-1.22464679914735E-16,0.,-1.));
#6990=DIRECTION('center_axis',(0.,1.,0.));
#6991=DIRECTION('ref_axis',(0.,0.,1.));
#6992=DIRECTION('center_axis',(1.,0.,1.22464679914734E-16));
#6993=DIRECTION('ref_axis',(-6.12323399573672E-17,0.,1.));
#6994=DIRECTION('center_axis',(0.,-1.,0.));
#6995=DIRECTION('ref_axis',(6.12323399573672E-17,0.,-1.));
#6996=DIRECTION('center_axis',(0.,1.,0.));
#6997=DIRECTION('ref_axis',(0.,0.,1.));
#6998=DIRECTION('center_axis',(0.,1.,0.));
#6999=DIRECTION('ref_axis',(0.,0.,1.));
#7000=DIRECTION('center_axis',(0.,1.,0.));
#7001=DIRECTION('ref_axis',(0.,0.,1.));
#7002=DIRECTION('center_axis',(0.,-1.,0.));
#7003=DIRECTION('ref_axis',(0.,0.,-1.));
#7004=DIRECTION('center_axis',(0.707106781186549,0.707106781186546,-5.38036114367792E-17));
#7005=DIRECTION('ref_axis',(0.,0.,1.));
#7006=DIRECTION('center_axis',(0.707106781186549,0.707106781186546,-5.38036114367792E-17));
#7007=DIRECTION('ref_axis',(3.80448984992727E-17,3.80448984992726E-17,1.));
#7008=DIRECTION('center_axis',(-0.707106781186546,0.707106781186549,0.));
#7009=DIRECTION('ref_axis',(0.,0.,-1.));
#7010=DIRECTION('center_axis',(0.707106781186549,0.707106781186546,-5.38036114367792E-17));
#7011=DIRECTION('ref_axis',(3.80448984992727E-17,3.80448984992726E-17,1.));
#7012=DIRECTION('center_axis',(0.707106781186546,-0.707106781186549,1.22464679914734E-16));
#7013=DIRECTION('ref_axis',(0.,0.,1.));
#7014=DIRECTION('center_axis',(-0.707106781186549,-0.707106781186546,0.));
#7015=DIRECTION('ref_axis',(0.,0.,-1.));
#7016=DIRECTION('center_axis',(0.707106781186549,0.707106781186546,-5.38036114367792E-17));
#7017=DIRECTION('ref_axis',(3.80448984992727E-17,3.80448984992726E-17,1.));
#7018=DIRECTION('center_axis',(0.707106781186549,0.707106781186546,-5.38036114367792E-17));
#7019=DIRECTION('ref_axis',(3.80448984992727E-17,3.80448984992726E-17,1.));
#7020=DIRECTION('center_axis',(0.707106781186549,0.707106781186546,-5.38036114367792E-17));
#7021=DIRECTION('ref_axis',(1.29893408435324E-16,-5.38036114367791E-17,
1.));
#7022=DIRECTION('center_axis',(-0.707106781186549,-0.707106781186546,5.38036114367792E-17));
#7023=DIRECTION('ref_axis',(-1.29893408435324E-16,5.38036114367791E-17,
-1.));
#7024=DIRECTION('center_axis',(1.,-3.49148133884313E-15,-1.83697019872104E-16));
#7025=DIRECTION('ref_axis',(0.,-1.83697019872104E-16,1.));
#7026=DIRECTION('center_axis',(1.,-3.49148133884313E-15,-1.83697019872104E-16));
#7027=DIRECTION('ref_axis',(1.83697019872103E-16,-1.83697019872104E-16,
1.));
#7028=DIRECTION('center_axis',(3.49148133884313E-15,1.,3.06161699786841E-16));
#7029=DIRECTION('ref_axis',(0.,3.06161699786841E-16,-1.));
#7030=DIRECTION('center_axis',(1.,-3.49148133884313E-15,-1.83697019872104E-16));
#7031=DIRECTION('ref_axis',(1.83697019872103E-16,-1.83697019872104E-16,
1.));
#7032=DIRECTION('center_axis',(-3.71625375700952E-15,-1.,-6.12323399573671E-17));
#7033=DIRECTION('ref_axis',(0.,-1.22464679914734E-16,1.));
#7034=DIRECTION('center_axis',(-1.,3.71625375700953E-15,4.55109826834097E-31));
#7035=DIRECTION('ref_axis',(0.,1.22464679914733E-16,-1.));
#7036=DIRECTION('center_axis',(1.,-3.49148133884313E-15,-1.83697019872104E-16));
#7037=DIRECTION('ref_axis',(1.83697019872103E-16,-1.83697019872103E-16,
1.));
#7038=DIRECTION('center_axis',(1.,-3.49148133884313E-15,-1.83697019872104E-16));
#7039=DIRECTION('ref_axis',(1.83697019872103E-16,-1.83697019872103E-16,
1.));
#7040=DIRECTION('center_axis',(1.,-3.49148133884313E-15,-1.83697019872104E-16));
#7041=DIRECTION('ref_axis',(1.83697019872103E-16,-1.83697019872104E-16,
1.));
#7042=DIRECTION('center_axis',(-1.,3.49148133884313E-15,1.83697019872104E-16));
#7043=DIRECTION('ref_axis',(-1.83697019872103E-16,1.83697019872104E-16,
-1.));
#7044=DIRECTION('center_axis',(0.707106781186544,-0.707106781186551,-3.13590428307428E-16));
#7045=DIRECTION('ref_axis',(0.,-5.14716945902756E-16,1.));
#7046=DIRECTION('center_axis',(0.707106781186544,-0.707106781186551,-3.13590428307428E-16));
#7047=DIRECTION('ref_axis',(-4.73341490577976E-17,-4.90817985800547E-16,
1.));
#7048=DIRECTION('center_axis',(0.707106781186551,0.707106781186544,4.54949803549333E-16));
#7049=DIRECTION('ref_axis',(0.,6.43396182378445E-16,-1.));
#7050=DIRECTION('center_axis',(0.707106781186544,-0.707106781186551,-3.13590428307428E-16));
#7051=DIRECTION('ref_axis',(-4.73341490577977E-17,-4.90817985800548E-16,
1.));
#7052=DIRECTION('center_axis',(-0.707106781186551,-0.707106781186544,-3.05235227668501E-16));
#7053=DIRECTION('ref_axis',(0.,-6.19375626168253E-16,1.));
#7054=DIRECTION('center_axis',(-0.707106781186544,0.707106781186551,2.73727940853274E-16));
#7055=DIRECTION('ref_axis',(0.,3.87109766355158E-16,-1.));
#7056=DIRECTION('center_axis',(0.707106781186544,-0.707106781186551,-3.13590428307428E-16));
#7057=DIRECTION('ref_axis',(-9.1591177670555E-17,-5.35075014413304E-16,
1.));
#7058=DIRECTION('center_axis',(0.707106781186544,-0.707106781186551,-3.13590428307428E-16));
#7059=DIRECTION('ref_axis',(-9.1591177670555E-17,-5.35075014413304E-16,
1.));
#7060=DIRECTION('center_axis',(0.707106781186544,-0.707106781186551,-3.13590428307428E-16));
#7061=DIRECTION('ref_axis',(1.29893408435323E-16,-3.13590428307428E-16,
1.));
#7062=DIRECTION('center_axis',(-0.707106781186544,0.707106781186551,3.13590428307428E-16));
#7063=DIRECTION('ref_axis',(-1.29893408435323E-16,3.13590428307428E-16,
-1.));
#7064=DIRECTION('center_axis',(0.,-1.,-3.67394039744206E-16));
#7065=DIRECTION('ref_axis',(0.,0.,1.));
#7066=DIRECTION('center_axis',(0.,-1.,-3.67394039744206E-16));
#7067=DIRECTION('ref_axis',(0.,-3.67394039744206E-16,1.));
#7068=DIRECTION('center_axis',(1.,-4.49927934798557E-32,1.22464679914735E-16));
#7069=DIRECTION('ref_axis',(1.22464679914735E-16,6.43396182378445E-16,-1.));
#7070=DIRECTION('center_axis',(0.,-1.,-3.67394039744206E-16));
#7071=DIRECTION('ref_axis',(0.,-3.67394039744206E-16,1.));
#7072=DIRECTION('center_axis',(-1.,0.,1.22464679914734E-16));
#7073=DIRECTION('ref_axis',(6.12323399573672E-17,-6.19375626168253E-16,
1.));
#7074=DIRECTION('center_axis',(4.74072736285521E-32,1.,7.74219532710317E-16));
#7075=DIRECTION('ref_axis',(-6.12323399573672E-17,7.74219532710317E-16,
-1.));
#7076=DIRECTION('center_axis',(0.,-1.,-3.67394039744206E-16));
#7077=DIRECTION('ref_axis',(0.,-3.67394039744206E-16,1.));
#7078=DIRECTION('center_axis',(0.,-1.,-3.67394039744206E-16));
#7079=DIRECTION('ref_axis',(0.,-3.67394039744206E-16,1.));
#7080=DIRECTION('center_axis',(0.,-1.,-3.67394039744206E-16));
#7081=DIRECTION('ref_axis',(0.,-3.67394039744206E-16,1.));
#7082=DIRECTION('center_axis',(0.,1.,3.67394039744206E-16));
#7083=DIRECTION('ref_axis',(0.,3.67394039744206E-16,-1.));
#7084=DIRECTION('center_axis',(-0.707106781186554,-0.707106781186541,-3.13590428307426E-16));
#7085=DIRECTION('ref_axis',(0.,-5.14716945902756E-16,1.));
#7086=DIRECTION('center_axis',(-0.707106781186554,-0.707106781186541,-3.13590428307426E-16));
#7087=DIRECTION('ref_axis',(4.73341490577958E-17,-4.9081798580055E-16,1.));
#7088=DIRECTION('center_axis',(0.707106781186541,-0.707106781186554,-2.2747490177467E-16));
#7089=DIRECTION('ref_axis',(0.,3.21698091189223E-16,-1.));
#7090=DIRECTION('center_axis',(-0.707106781186554,-0.707106781186541,-3.13590428307426E-16));
#7091=DIRECTION('ref_axis',(4.73341490577959E-17,-4.9081798580055E-16,1.));
#7092=DIRECTION('center_axis',(-0.707106781186541,0.707106781186554,5.50164587497979E-16));
#7093=DIRECTION('ref_axis',(0.,-6.19375626168253E-16,1.));
#7094=DIRECTION('center_axis',(0.707106781186554,0.707106781186541,2.7372794085327E-16));
#7095=DIRECTION('ref_axis',(0.,3.87109766355158E-16,-1.));
#7096=DIRECTION('center_axis',(-0.707106781186554,-0.707106781186541,-3.13590428307426E-16));
#7097=DIRECTION('ref_axis',(9.15911776705531E-17,-5.35075014413308E-16,
1.));
#7098=DIRECTION('center_axis',(-0.707106781186554,-0.707106781186541,-3.13590428307426E-16));
#7099=DIRECTION('ref_axis',(9.15911776705531E-17,-5.35075014413308E-16,
1.));
#7100=DIRECTION('center_axis',(-0.707106781186554,-0.707106781186541,-3.13590428307426E-16));
#7101=DIRECTION('ref_axis',(-1.29893408435325E-16,-3.13590428307426E-16,
1.));
#7102=DIRECTION('center_axis',(0.707106781186554,0.707106781186541,3.13590428307426E-16));
#7103=DIRECTION('ref_axis',(1.29893408435325E-16,3.13590428307426E-16,-1.));
#7104=DIRECTION('center_axis',(-1.,1.04744440165294E-14,-1.83697019872101E-16));
#7105=DIRECTION('ref_axis',(0.,-1.83697019872098E-16,1.));
#7106=DIRECTION('center_axis',(-1.,1.04744440165294E-14,-1.83697019872101E-16));
#7107=DIRECTION('ref_axis',(-1.83697019872103E-16,-1.83697019872095E-16,
1.));
#7108=DIRECTION('center_axis',(-1.04744440165294E-14,-1.,-6.12323399573585E-17));
#7109=DIRECTION('ref_axis',(0.,6.12323399573585E-17,-1.));
#7110=DIRECTION('center_axis',(-1.,1.04744440165294E-14,-1.83697019872101E-16));
#7111=DIRECTION('ref_axis',(-1.83697019872103E-16,-1.83697019872095E-16,
1.));
#7112=DIRECTION('center_axis',(1.05293856448603E-14,1.,3.06161699786836E-16));
#7113=DIRECTION('ref_axis',(0.,-2.44929359829469E-16,1.));
#7114=DIRECTION('center_axis',(1.,-1.05293856448603E-14,-2.57895568539326E-30));
#7115=DIRECTION('ref_axis',(0.,2.44929359829472E-16,-1.));
#7116=DIRECTION('center_axis',(-1.,1.04744440165294E-14,-1.83697019872101E-16));
#7117=DIRECTION('ref_axis',(-1.83697019872103E-16,-1.83697019872103E-16,
1.));
#7118=DIRECTION('center_axis',(-1.,1.04744440165294E-14,-1.83697019872101E-16));
#7119=DIRECTION('ref_axis',(-1.83697019872103E-16,-1.83697019872103E-16,
1.));
#7120=DIRECTION('center_axis',(-1.,1.04744440165294E-14,-1.83697019872101E-16));
#7121=DIRECTION('ref_axis',(-1.83697019872103E-16,-1.83697019872101E-16,
1.));
#7122=DIRECTION('center_axis',(1.,-1.04744440165294E-14,1.83697019872101E-16));
#7123=DIRECTION('ref_axis',(1.83697019872103E-16,1.83697019872101E-16,-1.));
#7124=DIRECTION('center_axis',(-0.707106781186539,0.707106781186556,-5.38036114367774E-17));
#7125=DIRECTION('ref_axis',(0.,0.,1.));
#7126=DIRECTION('center_axis',(-0.707106781186539,0.707106781186556,-5.38036114367774E-17));
#7127=DIRECTION('ref_axis',(-3.80448984992709E-17,3.80448984992719E-17,
1.));
#7128=DIRECTION('center_axis',(-0.707106781186556,-0.707106781186539,0.));
#7129=DIRECTION('ref_axis',(0.,0.,-1.));
#7130=DIRECTION('center_axis',(-0.707106781186539,0.707106781186556,-5.38036114367774E-17));
#7131=DIRECTION('ref_axis',(-3.80448984992709E-17,3.80448984992719E-17,
1.));
#7132=DIRECTION('center_axis',(0.707106781186556,0.707106781186539,1.22464679914734E-16));
#7133=DIRECTION('ref_axis',(0.,0.,1.));
#7134=DIRECTION('center_axis',(0.707106781186539,-0.707106781186556,0.));
#7135=DIRECTION('ref_axis',(0.,0.,-1.));
#7136=DIRECTION('center_axis',(-0.707106781186539,0.707106781186556,-5.38036114367774E-17));
#7137=DIRECTION('ref_axis',(-3.80448984992709E-17,3.80448984992719E-17,
1.));
#7138=DIRECTION('center_axis',(-0.707106781186539,0.707106781186556,-5.38036114367774E-17));
#7139=DIRECTION('ref_axis',(-3.80448984992709E-17,3.80448984992719E-17,
1.));
#7140=DIRECTION('center_axis',(-0.707106781186539,0.707106781186556,-5.38036114367774E-17));
#7141=DIRECTION('ref_axis',(-1.29893408435322E-16,-5.38036114367772E-17,
1.));
#7142=DIRECTION('center_axis',(0.707106781186539,-0.707106781186556,5.38036114367774E-17));
#7143=DIRECTION('ref_axis',(1.29893408435322E-16,5.38036114367772E-17,-1.));
#7144=DIRECTION('center_axis',(0.,0.,-1.));
#7145=DIRECTION('ref_axis',(-1.,0.,0.));
#7146=DIRECTION('center_axis',(0.,0.,1.));
#7147=DIRECTION('ref_axis',(1.,0.,0.));
#7148=DIRECTION('',(0.,0.,-1.));
#7149=DIRECTION('center_axis',(0.,0.,1.));
#7150=DIRECTION('ref_axis',(1.,0.,0.));
#7151=DIRECTION('center_axis',(0.,0.,-1.));
#7152=DIRECTION('ref_axis',(-1.,0.,0.));
#7153=DIRECTION('center_axis',(0.,0.,1.));
#7154=DIRECTION('ref_axis',(1.,0.,0.));
#7155=DIRECTION('',(0.,0.,1.));
#7156=DIRECTION('center_axis',(0.,0.,1.));
#7157=DIRECTION('ref_axis',(1.,0.,0.));
#7158=DIRECTION('center_axis',(0.,0.,1.));
#7159=DIRECTION('ref_axis',(1.,0.,0.));
#7160=DIRECTION('center_axis',(0.,0.,1.));
#7161=DIRECTION('ref_axis',(1.,0.,0.));
#7162=DIRECTION('center_axis',(0.,1.83697019872103E-16,-1.));
#7163=DIRECTION('ref_axis',(0.,1.,1.5654552317848E-16));
#7164=DIRECTION('center_axis',(0.,1.83697019872103E-16,-1.));
#7165=DIRECTION('ref_axis',(0.,1.,1.83697019872103E-16));
#7166=DIRECTION('center_axis',(-1.,1.22464679914735E-16,2.24963967399279E-32));
#7167=DIRECTION('ref_axis',(-1.22464679914735E-16,-1.,-1.956819039731E-16));
#7168=DIRECTION('center_axis',(0.,-1.83697019872103E-16,1.));
#7169=DIRECTION('ref_axis',(0.,1.,1.83697019872103E-16));
#7170=DIRECTION('center_axis',(0.,-1.83697019872103E-16,1.));
#7171=DIRECTION('ref_axis',(0.,1.,1.83697019872103E-16));
#7172=DIRECTION('center_axis',(0.,1.83697019872103E-16,-1.));
#7173=DIRECTION('ref_axis',(0.,1.,1.93432686686053E-16));
#7174=DIRECTION('center_axis',(0.,1.83697019872103E-16,-1.));
#7175=DIRECTION('ref_axis',(0.,1.,1.83697019872103E-16));
#7176=DIRECTION('center_axis',(0.,1.83697019872103E-16,-1.));
#7177=DIRECTION('ref_axis',(0.,1.,1.83697019872103E-16));
#7178=DIRECTION('center_axis',(-1.,1.22464679914735E-16,2.24963967399279E-32));
#7179=DIRECTION('ref_axis',(-1.22464679914735E-16,-1.,-1.6119390557171E-16));
#7180=DIRECTION('center_axis',(0.,-1.83697019872103E-16,1.));
#7181=DIRECTION('ref_axis',(0.,1.,1.83697019872103E-16));
#7182=DIRECTION('center_axis',(0.,-1.83697019872103E-16,1.));
#7183=DIRECTION('ref_axis',(0.,-1.,-1.83697019872103E-16));
#7184=DIRECTION('',(0.,1.83697019872103E-16,-1.));
#7185=DIRECTION('center_axis',(0.,-1.83697019872103E-16,1.));
#7186=DIRECTION('ref_axis',(0.,-1.,-1.83697019872103E-16));
#7187=DIRECTION('center_axis',(0.,-1.83697019872103E-16,1.));
#7188=DIRECTION('ref_axis',(0.,-1.,-1.83697019872103E-16));
#7189=DIRECTION('center_axis',(0.,1.83697019872103E-16,-1.));
#7190=DIRECTION('ref_axis',(0.,1.,1.83697019872103E-16));
#7191=DIRECTION('center_axis',(0.,-1.83697019872103E-16,1.));
#7192=DIRECTION('ref_axis',(0.,-1.,-1.83697019872103E-16));
#7193=DIRECTION('',(9.0785384304179E-17,0.741318920421686,0.671152932069007));
#7194=DIRECTION('center_axis',(0.,-1.83697019872103E-16,1.));
#7195=DIRECTION('ref_axis',(0.,-1.,-1.83697019872103E-16));
#7196=DIRECTION('center_axis',(0.,-1.83697019872103E-16,1.));
#7197=DIRECTION('ref_axis',(0.,-1.,-1.83697019872103E-16));
#7198=DIRECTION('',(-9.07853843041783E-17,0.741318920421681,0.671152932069013));
#7199=DIRECTION('center_axis',(0.,-1.83697019872103E-16,1.));
#7200=DIRECTION('ref_axis',(0.,-1.,-1.83697019872103E-16));
#7201=DIRECTION('center_axis',(0.,-1.83697019872103E-16,1.));
#7202=DIRECTION('ref_axis',(0.,-1.,-1.83697019872103E-16));
#7203=DIRECTION('',(0.,-1.83697019872103E-16,1.));
#7204=DIRECTION('center_axis',(0.,1.83697019872103E-16,-1.));
#7205=DIRECTION('ref_axis',(0.,1.,1.83697019872103E-16));
#7206=DIRECTION('center_axis',(0.,-1.83697019872103E-16,1.));
#7207=DIRECTION('ref_axis',(0.,-1.,-1.83697019872103E-16));
#7208=DIRECTION('center_axis',(0.,-1.83697019872103E-16,1.));
#7209=DIRECTION('ref_axis',(0.,-1.,-1.93432686686053E-16));
#7210=DIRECTION('center_axis',(0.,-1.83697019872103E-16,1.));
#7211=DIRECTION('ref_axis',(0.,-1.,-1.83697019872103E-16));
#7212=DIRECTION('center_axis',(-1.,-1.22464679914735E-16,-2.24963967399279E-32));
#7213=DIRECTION('ref_axis',(-1.22464679914735E-16,1.,1.6119390557171E-16));
#7214=DIRECTION('center_axis',(0.,1.83697019872103E-16,-1.));
#7215=DIRECTION('ref_axis',(0.,-1.,-1.83697019872103E-16));
#7216=DIRECTION('center_axis',(0.,-1.83697019872103E-16,1.));
#7217=DIRECTION('ref_axis',(0.,-1.,-1.5654552317848E-16));
#7218=DIRECTION('center_axis',(0.,-1.83697019872103E-16,1.));
#7219=DIRECTION('ref_axis',(0.,-1.,-1.83697019872103E-16));
#7220=DIRECTION('center_axis',(-1.,-1.22464679914735E-16,-2.24963967399279E-32));
#7221=DIRECTION('ref_axis',(-1.22464679914735E-16,1.,1.956819039731E-16));
#7222=DIRECTION('center_axis',(0.,1.83697019872103E-16,-1.));
#7223=DIRECTION('ref_axis',(0.,-1.,-1.83697019872103E-16));
#7224=DIRECTION('center_axis',(0.,-1.83697019872103E-16,1.));
#7225=DIRECTION('ref_axis',(0.,-1.,-1.83697019872103E-16));
#7226=DIRECTION('',(0.,-1.83697019872103E-16,1.));
#7227=DIRECTION('center_axis',(0.,-1.83697019872103E-16,1.));
#7228=DIRECTION('ref_axis',(0.,-1.,-1.83697019872103E-16));
#7229=DIRECTION('center_axis',(0.,-1.83697019872103E-16,1.));
#7230=DIRECTION('ref_axis',(0.,-1.,-1.83697019872103E-16));
#7231=DIRECTION('center_axis',(0.,1.83697019872103E-16,-1.));
#7232=DIRECTION('ref_axis',(0.,1.,1.83697019872103E-16));
#7233=DIRECTION('center_axis',(0.,-1.83697019872103E-16,1.));
#7234=DIRECTION('ref_axis',(0.,-1.,-1.83697019872103E-16));
#7235=DIRECTION('',(-9.07853843041785E-17,-0.741318920421682,-0.671152932069012));
#7236=DIRECTION('center_axis',(0.,-1.83697019872103E-16,1.));
#7237=DIRECTION('ref_axis',(0.,-1.,-1.83697019872103E-16));
#7238=DIRECTION('center_axis',(0.,-1.83697019872103E-16,1.));
#7239=DIRECTION('ref_axis',(0.,-1.,-1.83697019872103E-16));
#7240=DIRECTION('',(9.07853843041792E-17,-0.741318920421688,-0.671152932069005));
#7241=DIRECTION('center_axis',(0.,-1.83697019872103E-16,1.));
#7242=DIRECTION('ref_axis',(0.,-1.,-1.83697019872103E-16));
#7243=DIRECTION('center_axis',(0.,-1.83697019872103E-16,1.));
#7244=DIRECTION('ref_axis',(0.,-1.,-1.83697019872103E-16));
#7245=DIRECTION('',(0.,1.83697019872103E-16,-1.));
#7246=DIRECTION('center_axis',(0.,1.83697019872103E-16,-1.));
#7247=DIRECTION('ref_axis',(0.,1.,1.83697019872103E-16));
#7248=DIRECTION('center_axis',(0.,-1.83697019872103E-16,1.));
#7249=DIRECTION('ref_axis',(0.,-1.,-1.83697019872103E-16));
#8650=CARTESIAN_POINT('',(0.,0.,0.));
#8651=CARTESIAN_POINT('Origin',(0.,1.73472347597681E-15,-2.60208521396521E-15));
#8652=CARTESIAN_POINT('',(1.34711147906209E-15,11.,2.44444444444444));
#8653=CARTESIAN_POINT('Origin',(0.,5.61296449609204E-16,2.44444444444444));
#8654=CARTESIAN_POINT('',(-1.34711147906209E-15,11.,-2.44444444444444));
#8655=CARTESIAN_POINT('Origin',(-1.53080849893419E-15,12.5,-3.05872465563923E-16));
#8656=CARTESIAN_POINT('Origin',(0.,1.45937076898393E-15,-2.44444444444445));
#8657=CARTESIAN_POINT('Origin',(0.,-6.84346607882717E-31,5.5));
#8658=CARTESIAN_POINT('',(-9.18485099360515E-16,7.5,4.95));
#8659=CARTESIAN_POINT('Origin',(0.,1.01033360929656E-16,4.95));
#8660=CARTESIAN_POINT('',(-9.85840673313618E-16,8.04999999999999,5.50000000000001));
#8661=CARTESIAN_POINT('',(-9.85840673313618E-16,8.04999999999999,5.5));
#8662=CARTESIAN_POINT('Origin',(0.,-6.84346607882717E-31,5.5));
#8663=CARTESIAN_POINT('Origin',(0.,0.,5.5));
#8664=CARTESIAN_POINT('',(9.52162886337066E-16,-7.5,-4.95000000000001));
#8665=CARTESIAN_POINT('',(-9.18485099360515E-16,7.5,-4.95000000000001));
#8666=CARTESIAN_POINT('Origin',(0.,1.91963385766348E-15,-4.95000000000001));
#8667=CARTESIAN_POINT('Origin',(0.,1.91963385766348E-15,-4.95000000000001));
#8668=CARTESIAN_POINT('',(-9.18485099360515E-16,7.5,5.5));
#8669=CARTESIAN_POINT('Origin',(0.,1.91963385766348E-15,-4.95000000000001));
#8670=CARTESIAN_POINT('',(-9.85840673313618E-16,-8.04999999999999,-5.50000000000001));
#8671=CARTESIAN_POINT('',(-9.18485099360515E-16,-7.5,-4.95000000000001));
#8672=CARTESIAN_POINT('Origin',(0.,2.02066721859313E-15,-5.50000000000001));
#8673=CARTESIAN_POINT('Origin',(0.,0.,5.5));
#8674=CARTESIAN_POINT('',(-1.34711147906209E-15,11.,-5.50000000000001));
#8675=CARTESIAN_POINT('',(-1.34711147906209E-15,11.,5.5));
#8676=CARTESIAN_POINT('Origin',(0.,2.02066721859313E-15,-5.50000000000001));
#8677=CARTESIAN_POINT('Origin',(0.,0.,5.5));
#8678=CARTESIAN_POINT('',(-1.34711147906209E-15,11.,5.50000000000001));
#8679=CARTESIAN_POINT('Origin',(0.,-9.03463585147651E-31,5.50000000000001));
#8680=CARTESIAN_POINT('',(-1.34711147906209E-15,11.,5.5));
#8681=CARTESIAN_POINT('Origin',(0.,8.04999999999999,5.50000000000001));
#8682=CARTESIAN_POINT('Origin',(0.,8.04999999999999,-5.50000000000001));
#8683=CARTESIAN_POINT('Origin',(0.,12.5,0.));
#8684=CARTESIAN_POINT('',(-2.86797988869785,12.5,2.15064044727603E-32));
#8685=CARTESIAN_POINT('',(2.86797988869785,12.5,2.15064044727603E-32));
#8686=CARTESIAN_POINT('Origin',(0.,12.5,0.));
#8687=CARTESIAN_POINT('Origin',(0.,2.02066721859313E-15,-5.50000000000001));
#8688=CARTESIAN_POINT('',(-2.14313189850787E-15,17.5,-4.95000000000001));
#8689=CARTESIAN_POINT('Origin',(0.,1.91963385766348E-15,-4.95000000000001));
#8690=CARTESIAN_POINT('',(-2.07577632455476E-15,16.95,-5.5));
#8691=CARTESIAN_POINT('',(-2.07577632455476E-15,16.95,-5.50000000000001));
#8692=CARTESIAN_POINT('Origin',(0.,2.02066721859313E-15,-5.50000000000001));
#8693=CARTESIAN_POINT('Origin',(0.,0.,5.5));
#8694=CARTESIAN_POINT('',(-1.7145055188063E-15,14.,-5.50000000000001));
#8695=CARTESIAN_POINT('Origin',(0.,2.02066721859313E-15,-5.50000000000001));
#8696=CARTESIAN_POINT('',(-1.7145055188063E-15,14.,-2.44444444444444));
#8697=CARTESIAN_POINT('',(-1.71450551880629E-15,14.,5.5));
#8698=CARTESIAN_POINT('Origin',(0.,1.45937076898393E-15,-2.44444444444445));
#8699=CARTESIAN_POINT('Origin',(0.,1.73472347597681E-15,-2.60208521396521E-15));
#8700=CARTESIAN_POINT('',(-1.7145055188063E-15,14.,2.44444444444445));
#8701=CARTESIAN_POINT('Origin',(-1.53080849893419E-15,12.5,-3.05872465563923E-16));
#8702=CARTESIAN_POINT('Origin',(0.,5.61296449609204E-16,2.44444444444444));
#8703=CARTESIAN_POINT('Origin',(0.,0.,5.5));
#8704=CARTESIAN_POINT('',(-1.7145055188063E-15,14.,5.5));
#8705=CARTESIAN_POINT('',(-1.71450551880629E-15,14.,5.5));
#8706=CARTESIAN_POINT('Origin',(0.,7.91087864377601E-31,5.5));
#8707=CARTESIAN_POINT('Origin',(0.,1.01033360929657E-16,4.94999999999999));
#8708=CARTESIAN_POINT('',(2.14313189850787E-15,17.5,4.95));
#8709=CARTESIAN_POINT('',(-2.14313189850787E-15,-17.5,4.94999999999999));
#8710=CARTESIAN_POINT('Origin',(0.,1.01033360929657E-16,4.94999999999999));
#8711=CARTESIAN_POINT('',(-2.07577632455476E-15,-16.95,5.49999999999999));
#8712=CARTESIAN_POINT('',(-2.14313189850787E-15,-17.5,4.94999999999999));
#8713=CARTESIAN_POINT('Origin',(0.,1.2092979527909E-30,5.49999999999999));
#8714=CARTESIAN_POINT('Origin',(0.,1.01033360929657E-16,4.94999999999999));
#8715=CARTESIAN_POINT('Origin',(0.,0.,5.5));
#8716=CARTESIAN_POINT('',(-2.14313189850787E-15,17.5,5.5));
#8717=CARTESIAN_POINT('Origin',(0.,16.95,5.5));
#8718=CARTESIAN_POINT('Origin',(0.,16.95,-5.5));
#8719=CARTESIAN_POINT('Origin',(8.83883476483186,8.83883476483183,-6.7254514295974E-16));
#8720=CARTESIAN_POINT('',(6.81086673722698,10.8668027924367,-3.00013459892815E-16));
#8721=CARTESIAN_POINT('',(10.8668027924367,6.81086673722694,-1.04507682602666E-15));
#8722=CARTESIAN_POINT('Origin',(8.83883476483186,8.83883476483183,-6.7254514295974E-16));
#8723=CARTESIAN_POINT('Origin',(12.5,-4.36435167355392E-14,-2.2962127484013E-15));
#8724=CARTESIAN_POINT('',(12.5,2.86797988869781,-1.76937338979438E-15));
#8725=CARTESIAN_POINT('',(12.5,-2.86797988869789,-2.82305210700822E-15));
#8726=CARTESIAN_POINT('Origin',(12.5,-4.36435167355392E-14,-2.2962127484013E-15));
#8727=CARTESIAN_POINT('Origin',(8.8388347648318,-8.83883476483189,-3.91988035384285E-15));
#8728=CARTESIAN_POINT('',(10.8668027924367,-6.81086673722701,-3.54734867077593E-15));
#8729=CARTESIAN_POINT('',(6.8108667372269,-10.8668027924368,-4.29241203690977E-15));
#8730=CARTESIAN_POINT('Origin',(8.8388347648318,-8.83883476483189,-3.91988035384285E-15));
#8731=CARTESIAN_POINT('Origin',(0.,-12.5,-4.59242549680258E-15));
#8732=CARTESIAN_POINT('',(2.86797988869785,-12.5,-4.59242549680258E-15));
#8733=CARTESIAN_POINT('',(-2.86797988869785,-12.5,-4.59242549680258E-15));
#8734=CARTESIAN_POINT('Origin',(0.,-12.5,-4.59242549680258E-15));
#8735=CARTESIAN_POINT('Origin',(-8.83883476483192,-8.83883476483177,-3.91988035384282E-15));
#8736=CARTESIAN_POINT('',(-6.81086673722705,-10.8668027924367,-4.29241203690975E-15));
#8737=CARTESIAN_POINT('',(-10.8668027924368,-6.81086673722686,-3.54734867077589E-15));
#8738=CARTESIAN_POINT('Origin',(-8.83883476483192,-8.83883476483177,-3.91988035384282E-15));
#8739=CARTESIAN_POINT('Origin',(-12.5,1.30930550206618E-13,-2.29621274840126E-15));
#8740=CARTESIAN_POINT('',(-12.5,-2.86797988869772,-2.82305210700818E-15));
#8741=CARTESIAN_POINT('',(-12.5,2.86797988869798,-1.76937338979434E-15));
#8742=CARTESIAN_POINT('Origin',(-12.5,1.30930550206618E-13,-2.29621274840126E-15));
#8743=CARTESIAN_POINT('Origin',(-8.83883476483174,8.83883476483195,-6.72545142959718E-16));
#8744=CARTESIAN_POINT('',(-10.8668027924367,6.81086673722708,-1.04507682602664E-15));
#8745=CARTESIAN_POINT('',(-6.81086673722683,10.8668027924368,-3.00013459892799E-16));
#8746=CARTESIAN_POINT('Origin',(-8.83883476483174,8.83883476483195,-6.72545142959718E-16));
#8747=CARTESIAN_POINT('Origin',(0.,12.5,0.));
#8748=CARTESIAN_POINT('',(-3.94762635814864E-16,13.25,-3.22348154659542));
#8749=CARTESIAN_POINT('Origin',(0.,13.25,0.));
#8750=CARTESIAN_POINT('',(-3.94762635814864E-16,11.7500000000001,-3.22348154659542));
#8751=CARTESIAN_POINT('Origin',(-2.5740463218088E-16,12.5,-2.10186832938358));
#8752=CARTESIAN_POINT('Origin',(0.,11.7500000000001,0.));
#8753=CARTESIAN_POINT('Origin',(0.,12.5,-9.15066633577766E-14));
#8754=CARTESIAN_POINT('',(-2.86797988869795,12.5,-9.18578895968479E-14));
#8755=CARTESIAN_POINT('',(2.86797988869795,12.5,-9.15066633577766E-14));
#8756=CARTESIAN_POINT('Origin',(0.,12.5,-9.15066633577766E-14));
#8757=CARTESIAN_POINT('',(0.,11.7500000000001,2.7681778559145));
#8758=CARTESIAN_POINT('Origin',(0.,11.7500000000001,0.));
#8759=CARTESIAN_POINT('',(0.,13.25,2.7681778559145));
#8760=CARTESIAN_POINT('Origin',(0.,13.25,0.));
#8761=CARTESIAN_POINT('Origin',(0.,13.25,2.7681778559145));
#8762=CARTESIAN_POINT('Origin',(0.,11.7500000000001,3.22348154659542));
#8763=CARTESIAN_POINT('Origin',(8.83883476483188,8.83883476483185,-6.72545142959742E-16));
#8764=CARTESIAN_POINT('',(9.36916485072177,9.36916485072174,-3.22348154659542));
#8765=CARTESIAN_POINT('Origin',(9.36916485072177,9.36916485072174,-7.12897851537325E-16));
#8766=CARTESIAN_POINT('',(8.30850467894199,8.30850467894196,-3.22348154659542));
#8767=CARTESIAN_POINT('Origin',(8.83883476483188,8.83883476483185,-2.10186832938358));
#8768=CARTESIAN_POINT('Origin',(8.30850467894199,8.30850467894196,-6.32192434382159E-16));
#8769=CARTESIAN_POINT('Origin',(8.83883476483188,8.83883476483185,-9.21792085007363E-14));
#8770=CARTESIAN_POINT('',(6.81086673722692,10.8668027924368,-9.2354821620272E-14));
#8771=CARTESIAN_POINT('',(10.8668027924368,6.81086673722688,-9.2354821620272E-14));
#8772=CARTESIAN_POINT('Origin',(8.83883476483188,8.83883476483185,-9.21792085007363E-14));
#8773=CARTESIAN_POINT('',(8.30850467894199,8.30850467894196,2.7681778559145));
#8774=CARTESIAN_POINT('Origin',(8.30850467894199,8.30850467894196,-6.32192434382159E-16));
#8775=CARTESIAN_POINT('',(9.36916485072177,9.36916485072174,2.7681778559145));
#8776=CARTESIAN_POINT('Origin',(9.36916485072177,9.36916485072174,-7.12897851537325E-16));
#8777=CARTESIAN_POINT('Origin',(9.36916485072177,9.36916485072174,2.7681778559145));
#8778=CARTESIAN_POINT('Origin',(8.30850467894199,8.30850467894196,3.22348154659542));
#8779=CARTESIAN_POINT('Origin',(12.5,-4.36435167355393E-14,-2.2962127484013E-15));
#8780=CARTESIAN_POINT('',(13.25,-4.52752211501344E-14,-3.22348154659542));
#8781=CARTESIAN_POINT('Origin',(13.25,-4.62621277396715E-14,-2.43398551330537E-15));
#8782=CARTESIAN_POINT('',(11.7500000000001,-4.00379991418698E-14,-3.22348154659542));
#8783=CARTESIAN_POINT('Origin',(12.5,-4.30000051550871E-14,-2.10186832938358));
#8784=CARTESIAN_POINT('Origin',(11.7500000000001,-4.1024905731407E-14,-2.15843998349723E-15));
#8785=CARTESIAN_POINT('Origin',(12.5,-4.36435167355393E-14,-9.38028761061779E-14));
#8786=CARTESIAN_POINT('',(12.5,2.86797988869791,-9.36272629866423E-14));
#8787=CARTESIAN_POINT('',(12.5,-2.86797988869799,-9.43297154647848E-14));
#8788=CARTESIAN_POINT('Origin',(12.5,-4.36435167355393E-14,-9.38028761061779E-14));
#8789=CARTESIAN_POINT('',(11.7500000000001,-4.15334117540145E-14,2.7681778559145));
#8790=CARTESIAN_POINT('Origin',(11.7500000000001,-4.1024905731407E-14,-2.15843998349723E-15));
#8791=CARTESIAN_POINT('',(13.25,-4.6770633762279E-14,2.7681778559145));
#8792=CARTESIAN_POINT('Origin',(13.25,-4.62621277396715E-14,-2.43398551330537E-15));
#8793=CARTESIAN_POINT('Origin',(13.25,-4.6770633762279E-14,2.7681778559145));
#8794=CARTESIAN_POINT('Origin',(11.7500000000001,-4.16170496851293E-14,
3.22348154659542));
#8795=CARTESIAN_POINT('Origin',(8.83883476483182,-8.83883476483191,-3.91988035384286E-15));
#8796=CARTESIAN_POINT('',(9.36916485072171,-9.3691648507218,-3.22348154659542));
#8797=CARTESIAN_POINT('Origin',(9.36916485072171,-9.36916485072181,-4.15507317507342E-15));
#8798=CARTESIAN_POINT('',(8.30850467894193,-8.30850467894202,-3.22348154659542));
#8799=CARTESIAN_POINT('Origin',(8.83883476483182,-8.83883476483191,-2.10186832938358));
#8800=CARTESIAN_POINT('Origin',(8.30850467894193,-8.30850467894202,-3.68468753261229E-15));
#8801=CARTESIAN_POINT('Origin',(8.83883476483182,-8.83883476483191,-9.54265437116194E-14));
#8802=CARTESIAN_POINT('',(10.8668027924368,-6.81086673722696,-9.48171106018132E-14));
#8803=CARTESIAN_POINT('',(6.81086673722685,-10.8668027924369,-9.63872030604969E-14));
#8804=CARTESIAN_POINT('Origin',(8.83883476483182,-8.83883476483191,-9.54265437116194E-14));
#8805=CARTESIAN_POINT('',(8.30850467894193,-8.30850467894202,2.7681778559145));
#8806=CARTESIAN_POINT('Origin',(8.30850467894193,-8.30850467894202,-3.68468753261229E-15));
#8807=CARTESIAN_POINT('',(9.36916485072171,-9.36916485072181,2.7681778559145));
#8808=CARTESIAN_POINT('Origin',(9.36916485072171,-9.36916485072181,-4.15507317507342E-15));
#8809=CARTESIAN_POINT('Origin',(9.36916485072171,-9.36916485072181,2.7681778559145));
#8810=CARTESIAN_POINT('Origin',(8.30850467894193,-8.30850467894202,3.22348154659542));
#8811=CARTESIAN_POINT('Origin',(0.,-12.5,-4.59242549680259E-15));
#8812=CARTESIAN_POINT('',(3.94762635814864E-16,-13.25,-3.22348154659542));
#8813=CARTESIAN_POINT('Origin',(0.,-13.25,-4.86797102661073E-15));
#8814=CARTESIAN_POINT('',(3.94762635814864E-16,-11.7500000000001,-3.22348154659542));
#8815=CARTESIAN_POINT('Origin',(2.5740463218088E-16,-12.5,-2.10186832938358));
#8816=CARTESIAN_POINT('Origin',(0.,-11.7500000000001,-4.31687996699444E-15));
#8817=CARTESIAN_POINT('Origin',(0.,-12.5,-9.60990888545792E-14));
#8818=CARTESIAN_POINT('',(2.86797988869795,-12.5,-9.64503150936505E-14));
#8819=CARTESIAN_POINT('',(-2.86797988869795,-12.5,-9.60990888545792E-14));
#8820=CARTESIAN_POINT('Origin',(0.,-12.5,-9.60990888545792E-14));
#8821=CARTESIAN_POINT('',(0.,-11.7500000000001,2.7681778559145));
#8822=CARTESIAN_POINT('Origin',(0.,-11.7500000000001,-4.31687996699444E-15));
#8823=CARTESIAN_POINT('',(0.,-13.25,2.7681778559145));
#8824=CARTESIAN_POINT('Origin',(0.,-13.25,-4.86797102661073E-15));
#8825=CARTESIAN_POINT('Origin',(0.,-13.25,2.7681778559145));
#8826=CARTESIAN_POINT('Origin',(0.,-11.7500000000001,3.22348154659542));
#8827=CARTESIAN_POINT('Origin',(-8.83883476483194,-8.83883476483179,-3.91988035384283E-15));
#8828=CARTESIAN_POINT('',(-9.36916485072184,-9.36916485072167,-3.22348154659542));
#8829=CARTESIAN_POINT('Origin',(-9.36916485072184,-9.36916485072167,-4.15507317507339E-15));
#8830=CARTESIAN_POINT('',(-8.30850467894205,-8.3085046789419,-3.22348154659542));
#8831=CARTESIAN_POINT('Origin',(-8.83883476483194,-8.83883476483179,-2.10186832938358));
#8832=CARTESIAN_POINT('Origin',(-8.30850467894205,-8.3085046789419,-3.68468753261227E-15));
#8833=CARTESIAN_POINT('Origin',(-8.83883476483194,-8.83883476483179,-9.54265437116194E-14));
#8834=CARTESIAN_POINT('',(-6.810866737227,-10.8668027924368,-9.63872030604969E-14));
#8835=CARTESIAN_POINT('',(-10.8668027924369,-6.81086673722681,-9.48171106018132E-14));
#8836=CARTESIAN_POINT('Origin',(-8.83883476483194,-8.83883476483179,-9.54265437116194E-14));
#8837=CARTESIAN_POINT('',(-8.30850467894205,-8.3085046789419,2.7681778559145));
#8838=CARTESIAN_POINT('Origin',(-8.30850467894205,-8.3085046789419,-3.68468753261227E-15));
#8839=CARTESIAN_POINT('',(-9.36916485072184,-9.36916485072168,2.7681778559145));
#8840=CARTESIAN_POINT('Origin',(-9.36916485072184,-9.36916485072167,-4.15507317507339E-15));
#8841=CARTESIAN_POINT('Origin',(-9.36916485072184,-9.36916485072168,2.7681778559145));
#8842=CARTESIAN_POINT('Origin',(-8.30850467894205,-8.3085046789419,3.22348154659542));
#8843=CARTESIAN_POINT('Origin',(-12.5,1.30930550206618E-13,-2.29621274840127E-15));
#8844=CARTESIAN_POINT('',(-13.25,1.38983764536922E-13,-3.22348154659542));
#8845=CARTESIAN_POINT('Origin',(-13.25,1.38786383219015E-13,-2.43398551330534E-15));
#8846=CARTESIAN_POINT('',(-11.7500000000001,1.23272098512128E-13,-3.22348154659542));
#8847=CARTESIAN_POINT('Origin',(-12.5,1.31059252522708E-13,-2.10186832938358));
#8848=CARTESIAN_POINT('Origin',(-11.7500000000001,1.23074717194221E-13,
-2.1584399834972E-15));
#8849=CARTESIAN_POINT('Origin',(-12.5,1.30930550206618E-13,-9.38028761061778E-14));
#8850=CARTESIAN_POINT('',(-12.5,-2.86797988869782,-9.46809417038561E-14));
#8851=CARTESIAN_POINT('',(-12.5,2.86797988869808,-9.32760367475709E-14));
#8852=CARTESIAN_POINT('Origin',(-12.5,1.30930550206618E-13,-9.38028761061778E-14));
#8853=CARTESIAN_POINT('',(-11.7500000000001,1.22566211171614E-13,2.7681778559145));
#8854=CARTESIAN_POINT('Origin',(-11.7500000000001,1.23074717194221E-13,
-2.1584399834972E-15));
#8855=CARTESIAN_POINT('',(-13.25,1.38277877196407E-13,2.7681778559145));
#8856=CARTESIAN_POINT('Origin',(-13.25,1.38786383219015E-13,-2.43398551330534E-15));
#8857=CARTESIAN_POINT('Origin',(-13.25,1.38277877196407E-13,2.7681778559145));
#8858=CARTESIAN_POINT('Origin',(-11.7500000000001,1.22482573240499E-13,
3.22348154659542));
#8859=CARTESIAN_POINT('Origin',(-8.83883476483176,8.83883476483197,-6.72545142959719E-16));
#8860=CARTESIAN_POINT('',(-9.36916485072164,9.36916485072187,-3.22348154659542));
#8861=CARTESIAN_POINT('Origin',(-9.36916485072164,9.36916485072187,-7.12897851537301E-16));
#8862=CARTESIAN_POINT('',(-8.30850467894187,8.30850467894208,-3.22348154659542));
#8863=CARTESIAN_POINT('Origin',(-8.83883476483176,8.83883476483197,-2.10186832938358));
#8864=CARTESIAN_POINT('Origin',(-8.30850467894187,8.30850467894208,-6.32192434382138E-16));
#8865=CARTESIAN_POINT('Origin',(-8.83883476483176,8.83883476483197,-9.21792085007363E-14));
#8866=CARTESIAN_POINT('',(-10.8668027924367,6.81086673722703,-9.2354821620272E-14));
#8867=CARTESIAN_POINT('',(-6.81086673722677,10.8668027924369,-9.2354821620272E-14));
#8868=CARTESIAN_POINT('Origin',(-8.83883476483176,8.83883476483197,-9.21792085007363E-14));
#8869=CARTESIAN_POINT('',(-8.30850467894187,8.30850467894208,2.7681778559145));
#8870=CARTESIAN_POINT('Origin',(-8.30850467894187,8.30850467894208,-6.32192434382138E-16));
#8871=CARTESIAN_POINT('',(-9.36916485072164,9.36916485072187,2.7681778559145));
#8872=CARTESIAN_POINT('Origin',(-9.36916485072164,9.36916485072187,-7.12897851537301E-16));
#8873=CARTESIAN_POINT('Origin',(-9.36916485072164,9.36916485072187,2.7681778559145));
#8874=CARTESIAN_POINT('Origin',(-8.30850467894187,8.30850467894208,3.22348154659542));
#8875=CARTESIAN_POINT('Origin',(0.,0.,0.916666666666667));
#8876=CARTESIAN_POINT('',(12.5,-1.53080849893419E-15,0.916666666666667));
#8877=CARTESIAN_POINT('Origin',(0.,0.,0.916666666666667));
#8878=CARTESIAN_POINT('',(12.5,-1.53080849893419E-15,-0.916666666666667));
#8879=CARTESIAN_POINT('',(12.5,-1.53080849893419E-15,0.916666666666667));
#8880=CARTESIAN_POINT('Origin',(0.,0.,-0.916666666666667));
#8881=CARTESIAN_POINT('Origin',(0.,0.,0.916666666666667));
#8882=CARTESIAN_POINT('',(13.25,-1.62265700887024E-15,-0.916666666666667));
#8883=CARTESIAN_POINT('Origin',(0.,0.,-0.916666666666667));
#8884=CARTESIAN_POINT('',(13.25,-1.62265700887024E-15,0.916666666666667));
#8885=CARTESIAN_POINT('',(13.25,-1.62265700887024E-15,0.916666666666667));
#8886=CARTESIAN_POINT('Origin',(0.,0.,0.916666666666667));
#8887=CARTESIAN_POINT('Origin',(0.,0.,0.916666666666667));
#8888=CARTESIAN_POINT('Origin',(0.,0.,-0.916666666666667));
#8889=CARTESIAN_POINT('Origin',(0.,1.12259289921848E-17,5.43888888888889));
#8890=CARTESIAN_POINT('',(-1.38214998470436E-15,-11.2861111111111,5.49999999999999));
#8891=CARTESIAN_POINT('Origin',(0.,7.71876610523947E-31,5.5));
#8892=CARTESIAN_POINT('',(-1.3746660320429E-15,-11.225,5.43888888888889));
#8893=CARTESIAN_POINT('Origin',(-1.38214998470436E-15,-11.2861111111111,
5.43888888888889));
#8894=CARTESIAN_POINT('',(1.3746660320429E-15,11.225,5.43888888888889));
#8895=CARTESIAN_POINT('Origin',(0.,1.12259289921847E-17,5.43888888888889));
#8896=CARTESIAN_POINT('Origin',(0.,1.12259289921847E-17,5.43888888888889));
#8897=CARTESIAN_POINT('Origin',(0.,1.12259289921848E-17,5.43888888888889));
#8898=CARTESIAN_POINT('',(1.68695096582548E-15,13.775,5.43888888888889));
#8899=CARTESIAN_POINT('',(-1.68695096582548E-15,-13.775,5.43888888888889));
#8900=CARTESIAN_POINT('Origin',(0.,1.12259289921848E-17,5.43888888888889));
#8901=CARTESIAN_POINT('Origin',(0.,1.12259289921848E-17,5.43888888888889));
#8902=CARTESIAN_POINT('',(-1.67946701316402E-15,-13.7138888888889,5.49999999999999));
#8903=CARTESIAN_POINT('Origin',(-1.67946701316402E-15,-13.7138888888889,
5.43888888888889));
#8904=CARTESIAN_POINT('Origin',(0.,7.71876610523947E-31,5.5));
#8905=CARTESIAN_POINT('Origin',(0.,0.,5.5));
#8906=CARTESIAN_POINT('',(-1.68695096582548E-15,13.775,5.09259259259259));
#8907=CARTESIAN_POINT('',(-1.68695096582548E-15,13.775,5.5));
#8908=CARTESIAN_POINT('',(1.70072824231589E-15,-13.775,5.09259259259259));
#8909=CARTESIAN_POINT('Origin',(0.,7.48395266145613E-17,5.09259259259259));
#8910=CARTESIAN_POINT('Origin',(0.,7.48395266145613E-17,5.09259259259259));
#8911=CARTESIAN_POINT('Origin',(0.,1.12259289921841E-16,4.88888888888888));
#8912=CARTESIAN_POINT('',(-1.7145055188063E-15,-14.,4.88888888888888));
#8913=CARTESIAN_POINT('Origin',(0.,1.12259289921841E-16,4.88888888888888));
#8914=CARTESIAN_POINT('',(-1.71450551880629E-15,-14.,4.88888888888888));
#8915=CARTESIAN_POINT('Origin',(0.,7.4839526614561E-17,5.09259259259259));
#8916=CARTESIAN_POINT('',(-1.34711147906209E-15,11.,4.88888888888889));
#8917=CARTESIAN_POINT('Origin',(0.,1.12259289921842E-16,4.88888888888888));
#8918=CARTESIAN_POINT('',(-1.3746660320429E-15,11.225,5.09259259259259));
#8919=CARTESIAN_POINT('',(-1.3746660320429E-15,11.225,5.09259259259259));
#8920=CARTESIAN_POINT('Origin',(0.,7.4839526614561E-17,5.09259259259259));
#8921=CARTESIAN_POINT('Origin',(0.,0.,5.5));
#8922=CARTESIAN_POINT('',(-1.3746660320429E-15,11.225,5.5));
#8923=CARTESIAN_POINT('Origin',(0.,13.775,5.5));
#8924=CARTESIAN_POINT('Origin',(0.,14.,4.88888888888889));
#8925=CARTESIAN_POINT('Origin',(0.,2.00944128960095E-15,-5.43888888888889));
#8926=CARTESIAN_POINT('',(-1.68695096582548E-15,13.775,-5.43888888888889));
#8927=CARTESIAN_POINT('Origin',(0.,2.00944128960095E-15,-5.4388888888889));
#8928=CARTESIAN_POINT('',(-1.67946701316402E-15,13.7138888888889,-5.5));
#8929=CARTESIAN_POINT('Origin',(-1.67946701316402E-15,13.7138888888889,
-5.43888888888889));
#8930=CARTESIAN_POINT('Origin',(0.,2.02066721859313E-15,-5.50000000000001));
#8931=CARTESIAN_POINT('Origin',(0.,2.00944128960095E-15,-5.43888888888889));
#8932=CARTESIAN_POINT('',(-1.38214998470436E-15,11.2861111111111,-5.5));
#8933=CARTESIAN_POINT('Origin',(0.,2.02066721859313E-15,-5.50000000000001));
#8934=CARTESIAN_POINT('',(-1.3746660320429E-15,11.225,-5.43888888888889));
#8935=CARTESIAN_POINT('Origin',(-1.38214998470436E-15,11.2861111111111,
-5.43888888888889));
#8936=CARTESIAN_POINT('Origin',(0.,2.00944128960095E-15,-5.43888888888889));
#8937=CARTESIAN_POINT('Origin',(0.,0.,5.5));
#8938=CARTESIAN_POINT('',(-1.3746660320429E-15,11.225,-5.0925925925926));
#8939=CARTESIAN_POINT('',(-1.3746660320429E-15,11.225,5.5));
#8940=CARTESIAN_POINT('',(1.3746660320429E-15,-11.225,-5.0925925925926));
#8941=CARTESIAN_POINT('Origin',(0.,1.94582769197857E-15,-5.0925925925926));
#8942=CARTESIAN_POINT('Origin',(0.,1.94582769197857E-15,-5.0925925925926));
#8943=CARTESIAN_POINT('Origin',(0.,1.90840792867129E-15,-4.88888888888889));
#8944=CARTESIAN_POINT('',(-1.34711147906209E-15,-11.,-4.8888888888889));
#8945=CARTESIAN_POINT('Origin',(0.,1.90840792867129E-15,-4.88888888888889));
#8946=CARTESIAN_POINT('',(-1.34711147906209E-15,-11.,-4.88888888888889));
#8947=CARTESIAN_POINT('Origin',(0.,1.94582769197857E-15,-5.0925925925926));
#8948=CARTESIAN_POINT('',(-1.7145055188063E-15,14.,-4.88888888888889));
#8949=CARTESIAN_POINT('Origin',(0.,1.90840792867129E-15,-4.88888888888889));
#8950=CARTESIAN_POINT('',(-1.68695096582548E-15,13.775,-5.09259259259259));
#8951=CARTESIAN_POINT('',(-1.68695096582548E-15,13.775,-5.0925925925926));
#8952=CARTESIAN_POINT('Origin',(0.,1.94582769197857E-15,-5.0925925925926));
#8953=CARTESIAN_POINT('Origin',(0.,0.,5.5));
#8954=CARTESIAN_POINT('',(-1.68695096582548E-15,13.775,5.5));
#8955=CARTESIAN_POINT('Origin',(0.,11.,-4.88888888888889));
#8956=CARTESIAN_POINT('Origin',(0.,13.775,-5.5));
#9483=UNCERTAINTY_MEASURE_WITH_UNIT(LENGTH_MEASURE(0.01),#9497,
'DISTANCE_ACCURACY_VALUE',
'Maximum model space distance between geometric entities at asserted c
onnectivities');
#9485=UNCERTAINTY_MEASURE_WITH_UNIT(LENGTH_MEASURE(0.01),#9497,
'DISTANCE_ACCURACY_VALUE',
'Maximum model space distance between geometric entities at asserted c
onnectivities');
#9494=(
GEOMETRIC_REPRESENTATION_CONTEXT(3)
GLOBAL_UNCERTAINTY_ASSIGNED_CONTEXT((#9483))
GLOBAL_UNIT_ASSIGNED_CONTEXT((#9497,#9499,#9500))
REPRESENTATION_CONTEXT('','3D')
);
#9496=(
GEOMETRIC_REPRESENTATION_CONTEXT(3)
GLOBAL_UNCERTAINTY_ASSIGNED_CONTEXT((#9485))
GLOBAL_UNIT_ASSIGNED_CONTEXT((#9497,#9499,#9500))
REPRESENTATION_CONTEXT('','3D')
);
#9497=(
LENGTH_UNIT()
NAMED_UNIT(*)
SI_UNIT(.MILLI.,.METRE.)
);
#9499=(
NAMED_UNIT(*)
PLANE_ANGLE_UNIT()
SI_UNIT($,.RADIAN.)
);
#9500=(
NAMED_UNIT(*)
SI_UNIT($,.STERADIAN.)
SOLID_ANGLE_UNIT()
);
#9509=SHAPE_DEFINITION_REPRESENTATION(#9519,#9546);
#9519=PRODUCT_DEFINITION_SHAPE('',$,#9557);
#9546=SHAPE_REPRESENTATION('',(#5576),#9494);
#9548=PRODUCT_DEFINITION_CONTEXT('part definition',#9580,'design');
#9557=PRODUCT_DEFINITION('Ball Bearing - Large','Ball Bearing - Large',
#9567,#9548);
#9567=PRODUCT_DEFINITION_FORMATION('',$,#9590);
#9580=APPLICATION_CONTEXT(
'Core Data for Automotive Mechanical Design Process');
#9581=PRODUCT_CONTEXT('part definition',#9580,'mechanical');
#9590=PRODUCT('Ball Bearing - Large','Ball Bearing - Large',$,(#9581));
#9594=PRESENTATION_STYLE_ASSIGNMENT((#9597));
#9597=SURFACE_STYLE_USAGE(.BOTH.,#9600);
#9600=SURFACE_SIDE_STYLE('',(#9603));
#9603=SURFACE_STYLE_FILL_AREA(#9606);
#9606=FILL_AREA_STYLE('Opaque(160,160,160)',(#9609));
#9609=FILL_AREA_STYLE_COLOUR('Opaque(160,160,160)',#9612);
#9612=COLOUR_RGB('Opaque(160,160,160)', 0.40784314, 0.44705882, 0.49803922);
ENDSEC;
END-ISO-10303-21;
